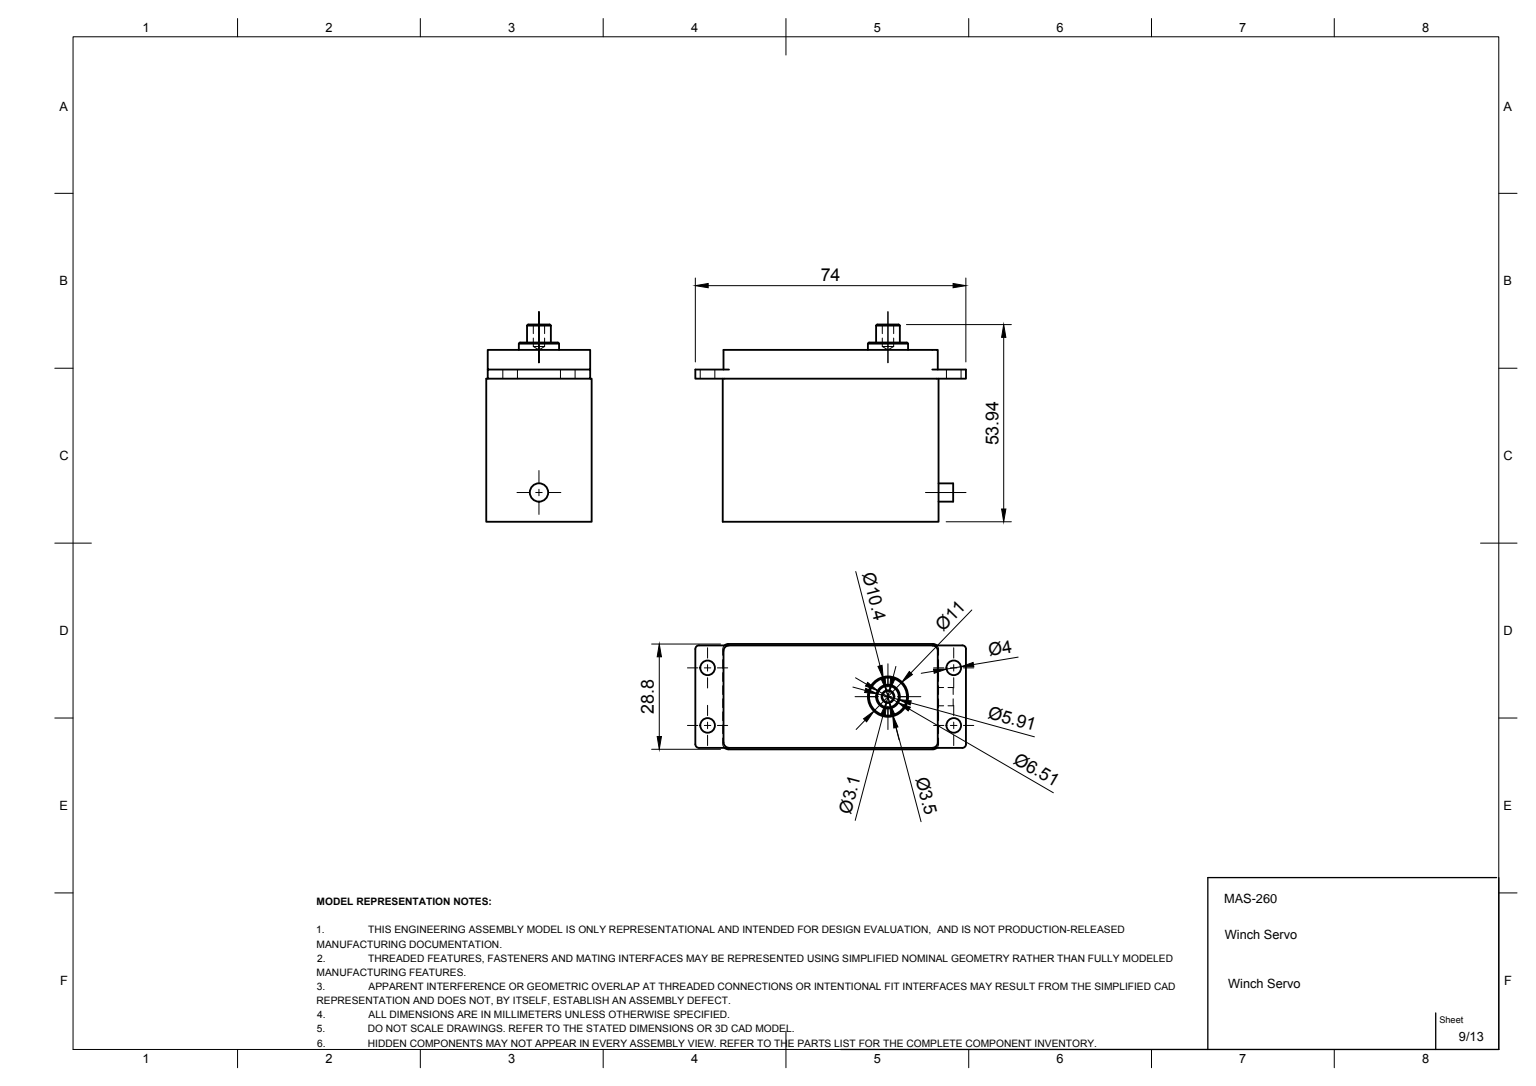
ISO-10303-21;
HEADER;
/* Generated by software containing ST-Developer
 * from STEP Tools, Inc. (www.steptools.com) 
 */

FILE_DESCRIPTION(
/* description */ (''),
/* implementation_level */ '2;1');

FILE_NAME(
/* name */ 'Winch Servo.step',
/* time_stamp */ '2026-10-15T13:29:10-07:00',
/* author */ (''),
/* organization */ (''),
/* preprocessor_version */ 'ST-DEVELOPER v20.2',
/* originating_system */ 'Autodesk Translation Framework v15.15.0.0',
/* authorisation */ '');

FILE_SCHEMA (('AUTOMOTIVE_DESIGN { 1 0 10303 214 3 1 1 }'));
ENDSEC;

DATA;
#10=MECHANICAL_DESIGN_GEOMETRIC_PRESENTATION_REPRESENTATION('',(#935),#83219);
#907=SHAPE_REPRESENTATION_RELATIONSHIP('SRR','None',#83302,#921);
#921=ADVANCED_BREP_SHAPE_REPRESENTATION('',(#949),#83207);
#935=STYLED_ITEM('',(#83381),#949);
#949=MANIFOLD_SOLID_BREP('Body1',#26931);
#1001=FACE_BOUND('',#3951,.T.);
#1002=FACE_BOUND('',#3957,.T.);
#1003=FACE_BOUND('',#3966,.T.);
#1004=FACE_BOUND('',#3968,.T.);
#1005=FACE_BOUND('',#3969,.T.);
#1006=FACE_BOUND('',#3971,.T.);
#1007=FACE_BOUND('',#3972,.T.);
#1008=FACE_BOUND('',#3974,.T.);
#1009=FACE_BOUND('',#3975,.T.);
#1010=FACE_BOUND('',#3985,.T.);
#1011=FACE_BOUND('',#3986,.T.);
#1012=FACE_BOUND('',#3993,.T.);
#1227=PLANE('',#27364);
#1228=PLANE('',#27382);
#1229=PLANE('',#27392);
#1230=PLANE('',#27395);
#1231=PLANE('',#27402);
#1232=PLANE('',#27409);
#1233=PLANE('',#27410);
#1234=PLANE('',#27413);
#1235=PLANE('',#27416);
#1236=PLANE('',#27421);
#1237=PLANE('',#27423);
#1238=PLANE('',#27426);
#1239=PLANE('',#27429);
#1240=PLANE('',#27431);
#1241=PLANE('',#27434);
#1242=PLANE('',#27437);
#1243=PLANE('',#27441);
#1244=PLANE('',#27445);
#1245=PLANE('',#27448);
#1246=PLANE('',#27451);
#1247=PLANE('',#27452);
#2173=CYLINDRICAL_SURFACE('',#27361,2.5);
#2174=CYLINDRICAL_SURFACE('',#27365,2.);
#2175=CYLINDRICAL_SURFACE('',#27368,2.);
#2176=CYLINDRICAL_SURFACE('',#27371,2.);
#2177=CYLINDRICAL_SURFACE('',#27374,2.);
#2178=CYLINDRICAL_SURFACE('',#27380,1.55);
#2179=CYLINDRICAL_SURFACE('',#27385,3.255);
#2180=CYLINDRICAL_SURFACE('',#27389,5.5);
#2181=CYLINDRICAL_SURFACE('',#27396,1.5);
#2182=CYLINDRICAL_SURFACE('',#27399,1.5);
#2183=CYLINDRICAL_SURFACE('',#27403,1.5);
#2184=CYLINDRICAL_SURFACE('',#27406,1.49999999999999);
#2185=CYLINDRICAL_SURFACE('',#27422,0.999999999999992);
#2186=CYLINDRICAL_SURFACE('',#27424,1.);
#2187=CYLINDRICAL_SURFACE('',#27427,0.999999999999999);
#2188=CYLINDRICAL_SURFACE('',#27430,0.999999999999996);
#2189=CYLINDRICAL_SURFACE('',#27438,1.5);
#2190=CYLINDRICAL_SURFACE('',#27442,1.5);
#2191=CYLINDRICAL_SURFACE('',#27446,1.5);
#2192=CYLINDRICAL_SURFACE('',#27449,1.49999999999999);
#2523=FACE_OUTER_BOUND('',#3942,.T.);
#2524=FACE_OUTER_BOUND('',#3943,.T.);
#2525=FACE_OUTER_BOUND('',#3944,.T.);
#2526=FACE_OUTER_BOUND('',#3945,.T.);
#2527=FACE_OUTER_BOUND('',#3946,.T.);
#2528=FACE_OUTER_BOUND('',#3947,.T.);
#2529=FACE_OUTER_BOUND('',#3948,.T.);
#2530=FACE_OUTER_BOUND('',#3949,.T.);
#2531=FACE_OUTER_BOUND('',#3950,.T.);
#2532=FACE_OUTER_BOUND('',#3952,.T.);
#2533=FACE_OUTER_BOUND('',#3953,.T.);
#2534=FACE_OUTER_BOUND('',#3954,.T.);
#2535=FACE_OUTER_BOUND('',#3955,.T.);
#2536=FACE_OUTER_BOUND('',#3956,.T.);
#2537=FACE_OUTER_BOUND('',#3958,.T.);
#2538=FACE_OUTER_BOUND('',#3959,.T.);
#2539=FACE_OUTER_BOUND('',#3960,.T.);
#2540=FACE_OUTER_BOUND('',#3961,.T.);
#2541=FACE_OUTER_BOUND('',#3962,.T.);
#2542=FACE_OUTER_BOUND('',#3963,.T.);
#2543=FACE_OUTER_BOUND('',#3964,.T.);
#2544=FACE_OUTER_BOUND('',#3965,.T.);
#2545=FACE_OUTER_BOUND('',#3967,.T.);
#2546=FACE_OUTER_BOUND('',#3970,.T.);
#2547=FACE_OUTER_BOUND('',#3973,.T.);
#2548=FACE_OUTER_BOUND('',#3976,.T.);
#2549=FACE_OUTER_BOUND('',#3977,.T.);
#2550=FACE_OUTER_BOUND('',#3978,.T.);
#2551=FACE_OUTER_BOUND('',#3979,.T.);
#2552=FACE_OUTER_BOUND('',#3980,.T.);
#2553=FACE_OUTER_BOUND('',#3981,.T.);
#2554=FACE_OUTER_BOUND('',#3982,.T.);
#2555=FACE_OUTER_BOUND('',#3983,.T.);
#2556=FACE_OUTER_BOUND('',#3984,.T.);
#2557=FACE_OUTER_BOUND('',#3987,.T.);
#2558=FACE_OUTER_BOUND('',#3988,.T.);
#2559=FACE_OUTER_BOUND('',#3989,.T.);
#2560=FACE_OUTER_BOUND('',#3990,.T.);
#2561=FACE_OUTER_BOUND('',#3991,.T.);
#2562=FACE_OUTER_BOUND('',#3992,.T.);
#2563=FACE_OUTER_BOUND('',#3994,.T.);
#2564=FACE_OUTER_BOUND('',#3995,.T.);
#2565=FACE_OUTER_BOUND('',#3996,.T.);
#2566=FACE_OUTER_BOUND('',#3997,.T.);
#2567=FACE_OUTER_BOUND('',#3998,.T.);
#3942=EDGE_LOOP('',(#18396,#18397,#18398,#18399));
#3943=EDGE_LOOP('',(#18400));
#3944=EDGE_LOOP('',(#18401,#18402,#18403,#18404));
#3945=EDGE_LOOP('',(#18405,#18406,#18407,#18408));
#3946=EDGE_LOOP('',(#18409,#18410,#18411,#18412));
#3947=EDGE_LOOP('',(#18413,#18414,#18415,#18416));
#3948=EDGE_LOOP('',(#18417,#18418,#18419,#18420));
#3949=EDGE_LOOP('',(#18421,#18422,#18423,#18424));
#3950=EDGE_LOOP('',(#18425));
#3951=EDGE_LOOP('',(#18426));
#3952=EDGE_LOOP('',(#18427,#18428,#18429));
#3953=EDGE_LOOP('',(#18430,#18431,#18432,#18433));
#3954=EDGE_LOOP('',(#18434,#18435,#18436,#18437));
#3955=EDGE_LOOP('',(#18438,#18439,#18440,#18441));
#3956=EDGE_LOOP('',(#18442));
#3957=EDGE_LOOP('',(#18443));
#3958=EDGE_LOOP('',(#18444,#18445,#18446,#18447));
#3959=EDGE_LOOP('',(#18448,#18449,#18450,#18451));
#3960=EDGE_LOOP('',(#18452,#18453,#18454,#18455));
#3961=EDGE_LOOP('',(#18456,#18457,#18458,#18459));
#3962=EDGE_LOOP('',(#18460,#18461,#18462,#18463));
#3963=EDGE_LOOP('',(#18464,#18465,#18466,#18467));
#3964=EDGE_LOOP('',(#18468,#18469,#18470,#18471));
#3965=EDGE_LOOP('',(#18472,#18473,#18474,#18475,#18476,#18477,#18478,#18479));
#3966=EDGE_LOOP('',(#18480));
#3967=EDGE_LOOP('',(#18481,#18482,#18483,#18484,#18485,#18486,#18487,#18488));
#3968=EDGE_LOOP('',(#18489));
#3969=EDGE_LOOP('',(#18490));
#3970=EDGE_LOOP('',(#18491,#18492,#18493,#18494,#18495,#18496,#18497,#18498));
#3971=EDGE_LOOP('',(#18499));
#3972=EDGE_LOOP('',(#18500));
#3973=EDGE_LOOP('',(#18501,#18502,#18503,#18504,#18505,#18506,#18507,#18508));
#3974=EDGE_LOOP('',(#18509));
#3975=EDGE_LOOP('',(#18510));
#3976=EDGE_LOOP('',(#18511,#18512,#18513,#18514));
#3977=EDGE_LOOP('',(#18515,#18516,#18517,#18518));
#3978=EDGE_LOOP('',(#18519,#18520,#18521,#18522,#18523,#18524,#18525,#18526,
#18527,#18528));
#3979=EDGE_LOOP('',(#18529,#18530,#18531,#18532));
#3980=EDGE_LOOP('',(#18533,#18534,#18535,#18536));
#3981=EDGE_LOOP('',(#18537,#18538,#18539,#18540));
#3982=EDGE_LOOP('',(#18541,#18542,#18543,#18544,#18545,#18546,#18547,#18548,
#18549,#18550));
#3983=EDGE_LOOP('',(#18551,#18552,#18553,#18554));
#3984=EDGE_LOOP('',(#18555,#18556,#18557,#18558,#18559,#18560,#18561,#18562));
#3985=EDGE_LOOP('',(#18563));
#3986=EDGE_LOOP('',(#18564));
#3987=EDGE_LOOP('',(#18565,#18566,#18567,#18568));
#3988=EDGE_LOOP('',(#18569,#18570,#18571,#18572));
#3989=EDGE_LOOP('',(#18573,#18574,#18575,#18576,#18577));
#3990=EDGE_LOOP('',(#18578,#18579,#18580,#18581));
#3991=EDGE_LOOP('',(#18582,#18583,#18584,#18585,#18586));
#3992=EDGE_LOOP('',(#18587,#18588,#18589,#18590));
#3993=EDGE_LOOP('',(#18591));
#3994=EDGE_LOOP('',(#18592,#18593,#18594,#18595,#18596));
#3995=EDGE_LOOP('',(#18597,#18598,#18599,#18600));
#3996=EDGE_LOOP('',(#18601,#18602,#18603,#18604,#18605));
#3997=EDGE_LOOP('',(#18606,#18607,#18608,#18609));
#3998=EDGE_LOOP('',(#18610,#18611,#18612,#18613,#18614,#18615,#18616,#18617));
#5589=LINE('',#36906,#8100);
#5590=LINE('',#36913,#8101);
#5591=LINE('',#36919,#8102);
#5592=LINE('',#36925,#8103);
#5593=LINE('',#36931,#8104);
#5594=LINE('',#36937,#8105);
#5595=LINE('',#36941,#8106);
#5596=LINE('',#36948,#8107);
#5597=LINE('',#36953,#8108);
#5598=LINE('',#36956,#8109);
#5599=LINE('',#36961,#8110);
#5600=LINE('',#36967,#8111);
#5601=LINE('',#36971,#8112);
#5602=LINE('',#36973,#8113);
#5603=LINE('',#36975,#8114);
#5604=LINE('',#36976,#8115);
#5605=LINE('',#36982,#8116);
#5606=LINE('',#36988,#8117);
#5607=LINE('',#36991,#8118);
#5608=LINE('',#36994,#8119);
#5609=LINE('',#36996,#8120);
#5610=LINE('',#36997,#8121);
#5611=LINE('',#37003,#8122);
#5612=LINE('',#37008,#8123);
#5613=LINE('',#37011,#8124);
#5614=LINE('',#37012,#8125);
#5615=LINE('',#37015,#8126);
#5616=LINE('',#37019,#8127);
#5617=LINE('',#37022,#8128);
#5618=LINE('',#37025,#8129);
#5619=LINE('',#37029,#8130);
#5620=LINE('',#37032,#8131);
#5621=LINE('',#37038,#8132);
#5622=LINE('',#37042,#8133);
#5623=LINE('',#37046,#8134);
#5624=LINE('',#37049,#8135);
#5625=LINE('',#37051,#8136);
#5626=LINE('',#37052,#8137);
#5627=LINE('',#37054,#8138);
#5628=LINE('',#37057,#8139);
#5629=LINE('',#37059,#8140);
#5630=LINE('',#37060,#8141);
#5631=LINE('',#37064,#8142);
#5632=LINE('',#37067,#8143);
#5633=LINE('',#37068,#8144);
#5634=LINE('',#37072,#8145);
#5635=LINE('',#37075,#8146);
#5636=LINE('',#37076,#8147);
#5637=LINE('',#37077,#8148);
#5638=LINE('',#37084,#8149);
#5639=LINE('',#37089,#8150);
#5640=LINE('',#37094,#8151);
#5641=LINE('',#37095,#8152);
#5642=LINE('',#37096,#8153);
#5643=LINE('',#37102,#8154);
#5644=LINE('',#37105,#8155);
#5645=LINE('',#37107,#8156);
#5646=LINE('',#37108,#8157);
#5647=LINE('',#37113,#8158);
#5648=LINE('',#37116,#8159);
#5649=LINE('',#37117,#8160);
#5650=LINE('',#37121,#8161);
#5651=LINE('',#37124,#8162);
#5652=LINE('',#37125,#8163);
#8100=VECTOR('',#30097,2.5);
#8101=VECTOR('',#30106,2.);
#8102=VECTOR('',#30113,2.);
#8103=VECTOR('',#30120,2.);
#8104=VECTOR('',#30127,2.);
#8105=VECTOR('',#30134,1.65);
#8106=VECTOR('',#30139,1.55);
#8107=VECTOR('',#30148,1.55);
#8108=VECTOR('',#30153,3.255);
#8109=VECTOR('',#30158,3.105);
#8110=VECTOR('',#30163,5.5);
#8111=VECTOR('',#30172,5.35);
#8112=VECTOR('',#30175,10.);
#8113=VECTOR('',#30176,10.);
#8114=VECTOR('',#30177,10.);
#8115=VECTOR('',#30178,10.);
#8116=VECTOR('',#30185,10.);
#8117=VECTOR('',#30190,10.);
#8118=VECTOR('',#30193,10.);
#8119=VECTOR('',#30196,10.);
#8120=VECTOR('',#30197,10.);
#8121=VECTOR('',#30198,10.);
#8122=VECTOR('',#30205,10.);
#8123=VECTOR('',#30210,10.);
#8124=VECTOR('',#30215,10.);
#8125=VECTOR('',#30216,10.);
#8126=VECTOR('',#30219,10.);
#8127=VECTOR('',#30222,10.);
#8128=VECTOR('',#30225,10.);
#8129=VECTOR('',#30228,10.);
#8130=VECTOR('',#30231,10.);
#8131=VECTOR('',#30234,10.);
#8132=VECTOR('',#30239,10.);
#8133=VECTOR('',#30242,10.);
#8134=VECTOR('',#30245,10.);
#8135=VECTOR('',#30248,10.);
#8136=VECTOR('',#30251,10.);
#8137=VECTOR('',#30252,10.);
#8138=VECTOR('',#30255,10.);
#8139=VECTOR('',#30258,10.);
#8140=VECTOR('',#30259,10.);
#8141=VECTOR('',#30260,10.);
#8142=VECTOR('',#30265,10.);
#8143=VECTOR('',#30268,10.);
#8144=VECTOR('',#30269,10.);
#8145=VECTOR('',#30274,10.);
#8146=VECTOR('',#30277,10.);
#8147=VECTOR('',#30278,10.);
#8148=VECTOR('',#30279,10.);
#8149=VECTOR('',#30288,10.);
#8150=VECTOR('',#30293,10.);
#8151=VECTOR('',#30298,10.);
#8152=VECTOR('',#30299,10.);
#8153=VECTOR('',#30300,10.);
#8154=VECTOR('',#30307,10.);
#8155=VECTOR('',#30310,10.);
#8156=VECTOR('',#30311,10.);
#8157=VECTOR('',#30312,10.);
#8158=VECTOR('',#30319,10.);
#8159=VECTOR('',#30322,10.);
#8160=VECTOR('',#30323,10.);
#8161=VECTOR('',#30328,10.);
#8162=VECTOR('',#30331,10.);
#8163=VECTOR('',#30332,10.);
#10392=CIRCLE('',#27362,2.5);
#10393=CIRCLE('',#27363,2.5);
#10394=CIRCLE('',#27366,2.);
#10395=CIRCLE('',#27367,2.);
#10396=CIRCLE('',#27369,2.);
#10397=CIRCLE('',#27370,2.);
#10398=CIRCLE('',#27372,2.);
#10399=CIRCLE('',#27373,2.);
#10400=CIRCLE('',#27375,2.);
#10401=CIRCLE('',#27376,2.);
#10402=CIRCLE('',#27378,1.55);
#10403=CIRCLE('',#27379,1.75);
#10404=CIRCLE('',#27381,1.55);
#10405=CIRCLE('',#27383,2.955);
#10406=CIRCLE('',#27386,3.255);
#10407=CIRCLE('',#27387,3.255);
#10408=CIRCLE('',#27390,5.5);
#10409=CIRCLE('',#27391,5.5);
#10410=CIRCLE('',#27393,5.2);
#10411=CIRCLE('',#27397,1.5);
#10412=CIRCLE('',#27398,1.5);
#10413=CIRCLE('',#27400,1.5);
#10414=CIRCLE('',#27401,1.5);
#10415=CIRCLE('',#27404,1.5);
#10416=CIRCLE('',#27405,1.5);
#10417=CIRCLE('',#27407,1.49999999999999);
#10418=CIRCLE('',#27408,1.49999999999999);
#10419=CIRCLE('',#27411,0.999999999999992);
#10420=CIRCLE('',#27412,0.999999999999996);
#10421=CIRCLE('',#27414,0.999999999999999);
#10422=CIRCLE('',#27415,1.);
#10423=CIRCLE('',#27417,1.5);
#10424=CIRCLE('',#27418,1.49999999999999);
#10425=CIRCLE('',#27419,0.999999999999996);
#10426=CIRCLE('',#27420,0.999999999999992);
#10427=CIRCLE('',#27425,1.);
#10428=CIRCLE('',#27428,0.999999999999999);
#10429=CIRCLE('',#27432,1.5);
#10430=CIRCLE('',#27433,1.5);
#10431=CIRCLE('',#27435,1.49999999999999);
#10432=CIRCLE('',#27436,1.5);
#10433=CIRCLE('',#27439,1.5);
#10434=CIRCLE('',#27440,1.5);
#10435=CIRCLE('',#27443,1.5);
#10436=CIRCLE('',#27444,1.5);
#10437=CIRCLE('',#27447,1.5);
#10438=CIRCLE('',#27450,1.49999999999999);
#11298=VERTEX_POINT('',#36903);
#11299=VERTEX_POINT('',#36905);
#11300=VERTEX_POINT('',#36910);
#11301=VERTEX_POINT('',#36912);
#11302=VERTEX_POINT('',#36916);
#11303=VERTEX_POINT('',#36918);
#11304=VERTEX_POINT('',#36922);
#11305=VERTEX_POINT('',#36924);
#11306=VERTEX_POINT('',#36928);
#11307=VERTEX_POINT('',#36930);
#11308=VERTEX_POINT('',#36934);
#11309=VERTEX_POINT('',#36936);
#11310=VERTEX_POINT('',#36940);
#11311=VERTEX_POINT('',#36944);
#11312=VERTEX_POINT('',#36947);
#11313=VERTEX_POINT('',#36950);
#11314=VERTEX_POINT('',#36952);
#11315=VERTEX_POINT('',#36958);
#11316=VERTEX_POINT('',#36960);
#11317=VERTEX_POINT('',#36964);
#11318=VERTEX_POINT('',#36969);
#11319=VERTEX_POINT('',#36970);
#11320=VERTEX_POINT('',#36972);
#11321=VERTEX_POINT('',#36974);
#11322=VERTEX_POINT('',#36978);
#11323=VERTEX_POINT('',#36980);
#11324=VERTEX_POINT('',#36984);
#11325=VERTEX_POINT('',#36985);
#11326=VERTEX_POINT('',#36987);
#11327=VERTEX_POINT('',#36989);
#11328=VERTEX_POINT('',#36993);
#11329=VERTEX_POINT('',#36995);
#11330=VERTEX_POINT('',#36999);
#11331=VERTEX_POINT('',#37001);
#11332=VERTEX_POINT('',#37005);
#11333=VERTEX_POINT('',#37007);
#11334=VERTEX_POINT('',#37014);
#11335=VERTEX_POINT('',#37016);
#11336=VERTEX_POINT('',#37018);
#11337=VERTEX_POINT('',#37020);
#11338=VERTEX_POINT('',#37024);
#11339=VERTEX_POINT('',#37026);
#11340=VERTEX_POINT('',#37028);
#11341=VERTEX_POINT('',#37030);
#11342=VERTEX_POINT('',#37034);
#11343=VERTEX_POINT('',#37035);
#11344=VERTEX_POINT('',#37037);
#11345=VERTEX_POINT('',#37039);
#11346=VERTEX_POINT('',#37041);
#11347=VERTEX_POINT('',#37043);
#11348=VERTEX_POINT('',#37045);
#11349=VERTEX_POINT('',#37047);
#11350=VERTEX_POINT('',#37056);
#11351=VERTEX_POINT('',#37058);
#11352=VERTEX_POINT('',#37062);
#11353=VERTEX_POINT('',#37066);
#11354=VERTEX_POINT('',#37070);
#11355=VERTEX_POINT('',#37074);
#11356=VERTEX_POINT('',#37080);
#11357=VERTEX_POINT('',#37082);
#11358=VERTEX_POINT('',#37086);
#11359=VERTEX_POINT('',#37088);
#11360=VERTEX_POINT('',#37092);
#11361=VERTEX_POINT('',#37093);
#11362=VERTEX_POINT('',#37098);
#11363=VERTEX_POINT('',#37100);
#11364=VERTEX_POINT('',#37104);
#11365=VERTEX_POINT('',#37106);
#11366=VERTEX_POINT('',#37110);
#11367=VERTEX_POINT('',#37115);
#11368=VERTEX_POINT('',#37119);
#11369=VERTEX_POINT('',#37123);
#14059=EDGE_CURVE('',#11298,#11298,#10392,.T.);
#14060=EDGE_CURVE('',#11298,#11299,#5589,.T.);
#14061=EDGE_CURVE('',#11299,#11299,#10393,.T.);
#14062=EDGE_CURVE('',#11300,#11300,#10394,.T.);
#14063=EDGE_CURVE('',#11300,#11301,#5590,.T.);
#14064=EDGE_CURVE('',#11301,#11301,#10395,.T.);
#14065=EDGE_CURVE('',#11302,#11302,#10396,.T.);
#14066=EDGE_CURVE('',#11302,#11303,#5591,.T.);
#14067=EDGE_CURVE('',#11303,#11303,#10397,.T.);
#14068=EDGE_CURVE('',#11304,#11304,#10398,.T.);
#14069=EDGE_CURVE('',#11304,#11305,#5592,.T.);
#14070=EDGE_CURVE('',#11305,#11305,#10399,.T.);
#14071=EDGE_CURVE('',#11306,#11306,#10400,.T.);
#14072=EDGE_CURVE('',#11306,#11307,#5593,.T.);
#14073=EDGE_CURVE('',#11307,#11307,#10401,.T.);
#14074=EDGE_CURVE('',#11308,#11308,#10402,.T.);
#14075=EDGE_CURVE('',#11308,#11309,#5594,.T.);
#14076=EDGE_CURVE('',#11309,#11309,#10403,.T.);
#14077=EDGE_CURVE('',#11308,#11310,#5595,.T.);
#14078=EDGE_CURVE('',#11310,#11310,#10404,.T.);
#14079=EDGE_CURVE('',#11311,#11311,#10405,.T.);
#14080=EDGE_CURVE('',#11312,#11310,#5596,.T.);
#14081=EDGE_CURVE('',#11313,#11313,#10406,.T.);
#14082=EDGE_CURVE('',#11313,#11314,#5597,.T.);
#14083=EDGE_CURVE('',#11314,#11314,#10407,.T.);
#14084=EDGE_CURVE('',#11314,#11311,#5598,.T.);
#14085=EDGE_CURVE('',#11315,#11315,#10408,.T.);
#14086=EDGE_CURVE('',#11315,#11316,#5599,.T.);
#14087=EDGE_CURVE('',#11316,#11316,#10409,.T.);
#14088=EDGE_CURVE('',#11317,#11317,#10410,.T.);
#14089=EDGE_CURVE('',#11316,#11317,#5600,.T.);
#14090=EDGE_CURVE('',#11318,#11319,#5601,.T.);
#14091=EDGE_CURVE('',#11318,#11320,#5602,.T.);
#14092=EDGE_CURVE('',#11321,#11320,#5603,.T.);
#14093=EDGE_CURVE('',#11319,#11321,#5604,.T.);
#14094=EDGE_CURVE('',#11319,#11322,#10411,.T.);
#14095=EDGE_CURVE('',#11323,#11321,#10412,.T.);
#14096=EDGE_CURVE('',#11322,#11323,#5605,.T.);
#14097=EDGE_CURVE('',#11324,#11325,#10413,.T.);
#14098=EDGE_CURVE('',#11324,#11326,#5606,.T.);
#14099=EDGE_CURVE('',#11327,#11326,#10414,.T.);
#14100=EDGE_CURVE('',#11325,#11327,#5607,.T.);
#14101=EDGE_CURVE('',#11325,#11328,#5608,.T.);
#14102=EDGE_CURVE('',#11329,#11327,#5609,.T.);
#14103=EDGE_CURVE('',#11328,#11329,#5610,.T.);
#14104=EDGE_CURVE('',#11328,#11330,#10415,.T.);
#14105=EDGE_CURVE('',#11331,#11329,#10416,.T.);
#14106=EDGE_CURVE('',#11330,#11331,#5611,.T.);
#14107=EDGE_CURVE('',#11332,#11318,#10417,.T.);
#14108=EDGE_CURVE('',#11332,#11333,#5612,.T.);
#14109=EDGE_CURVE('',#11320,#11333,#10418,.T.);
#14110=EDGE_CURVE('',#11333,#11331,#5613,.T.);
#14111=EDGE_CURVE('',#11326,#11323,#5614,.T.);
#14112=EDGE_CURVE('',#11322,#11334,#5615,.T.);
#14113=EDGE_CURVE('',#11334,#11335,#10419,.T.);
#14114=EDGE_CURVE('',#11335,#11336,#5616,.T.);
#14115=EDGE_CURVE('',#11336,#11337,#10420,.T.);
#14116=EDGE_CURVE('',#11337,#11332,#5617,.T.);
#14117=EDGE_CURVE('',#11330,#11338,#5618,.T.);
#14118=EDGE_CURVE('',#11338,#11339,#10421,.T.);
#14119=EDGE_CURVE('',#11339,#11340,#5619,.T.);
#14120=EDGE_CURVE('',#11340,#11341,#10422,.T.);
#14121=EDGE_CURVE('',#11341,#11324,#5620,.T.);
#14122=EDGE_CURVE('',#11342,#11343,#10423,.T.);
#14123=EDGE_CURVE('',#11343,#11344,#5621,.T.);
#14124=EDGE_CURVE('',#11344,#11345,#10424,.T.);
#14125=EDGE_CURVE('',#11345,#11346,#5622,.T.);
#14126=EDGE_CURVE('',#11347,#11346,#10425,.T.);
#14127=EDGE_CURVE('',#11347,#11348,#5623,.T.);
#14128=EDGE_CURVE('',#11349,#11348,#10426,.T.);
#14129=EDGE_CURVE('',#11349,#11342,#5624,.T.);
#14130=EDGE_CURVE('',#11347,#11336,#5625,.T.);
#14131=EDGE_CURVE('',#11348,#11335,#5626,.T.);
#14132=EDGE_CURVE('',#11349,#11334,#5627,.T.);
#14133=EDGE_CURVE('',#11350,#11341,#5628,.T.);
#14134=EDGE_CURVE('',#11351,#11350,#5629,.T.);
#14135=EDGE_CURVE('',#11342,#11351,#5630,.T.);
#14136=EDGE_CURVE('',#11352,#11350,#10427,.T.);
#14137=EDGE_CURVE('',#11352,#11340,#5631,.T.);
#14138=EDGE_CURVE('',#11352,#11353,#5632,.T.);
#14139=EDGE_CURVE('',#11353,#11339,#5633,.T.);
#14140=EDGE_CURVE('',#11354,#11353,#10428,.T.);
#14141=EDGE_CURVE('',#11354,#11338,#5634,.T.);
#14142=EDGE_CURVE('',#11354,#11355,#5635,.T.);
#14143=EDGE_CURVE('',#11346,#11337,#5636,.T.);
#14144=EDGE_CURVE('',#11355,#11345,#5637,.T.);
#14145=EDGE_CURVE('',#11356,#11351,#10429,.T.);
#14146=EDGE_CURVE('',#11355,#11357,#10430,.T.);
#14147=EDGE_CURVE('',#11357,#11356,#5638,.T.);
#14148=EDGE_CURVE('',#11345,#11358,#10431,.T.);
#14149=EDGE_CURVE('',#11358,#11359,#5639,.T.);
#14150=EDGE_CURVE('',#11359,#11355,#10432,.T.);
#14151=EDGE_CURVE('',#11360,#11361,#5640,.T.);
#14152=EDGE_CURVE('',#11360,#11344,#5641,.T.);
#14153=EDGE_CURVE('',#11361,#11343,#5642,.T.);
#14154=EDGE_CURVE('',#11362,#11361,#10433,.T.);
#14155=EDGE_CURVE('',#11363,#11342,#10434,.T.);
#14156=EDGE_CURVE('',#11362,#11363,#5643,.T.);
#14157=EDGE_CURVE('',#11362,#11364,#5644,.T.);
#14158=EDGE_CURVE('',#11365,#11363,#5645,.T.);
#14159=EDGE_CURVE('',#11364,#11365,#5646,.T.);
#14160=EDGE_CURVE('',#11366,#11364,#10435,.T.);
#14161=EDGE_CURVE('',#11351,#11365,#10436,.T.);
#14162=EDGE_CURVE('',#11366,#11356,#5647,.T.);
#14163=EDGE_CURVE('',#11366,#11367,#5648,.T.);
#14164=EDGE_CURVE('',#11367,#11357,#5649,.T.);
#14165=EDGE_CURVE('',#11368,#11367,#10437,.T.);
#14166=EDGE_CURVE('',#11368,#11359,#5650,.T.);
#14167=EDGE_CURVE('',#11368,#11369,#5651,.T.);
#14168=EDGE_CURVE('',#11369,#11358,#5652,.T.);
#14169=EDGE_CURVE('',#11360,#11369,#10438,.T.);
#18396=ORIENTED_EDGE('',*,*,#14059,.F.);
#18397=ORIENTED_EDGE('',*,*,#14060,.T.);
#18398=ORIENTED_EDGE('',*,*,#14061,.F.);
#18399=ORIENTED_EDGE('',*,*,#14060,.F.);
#18400=ORIENTED_EDGE('',*,*,#14059,.T.);
#18401=ORIENTED_EDGE('',*,*,#14062,.F.);
#18402=ORIENTED_EDGE('',*,*,#14063,.T.);
#18403=ORIENTED_EDGE('',*,*,#14064,.F.);
#18404=ORIENTED_EDGE('',*,*,#14063,.F.);
#18405=ORIENTED_EDGE('',*,*,#14065,.F.);
#18406=ORIENTED_EDGE('',*,*,#14066,.T.);
#18407=ORIENTED_EDGE('',*,*,#14067,.F.);
#18408=ORIENTED_EDGE('',*,*,#14066,.F.);
#18409=ORIENTED_EDGE('',*,*,#14068,.F.);
#18410=ORIENTED_EDGE('',*,*,#14069,.T.);
#18411=ORIENTED_EDGE('',*,*,#14070,.F.);
#18412=ORIENTED_EDGE('',*,*,#14069,.F.);
#18413=ORIENTED_EDGE('',*,*,#14071,.F.);
#18414=ORIENTED_EDGE('',*,*,#14072,.T.);
#18415=ORIENTED_EDGE('',*,*,#14073,.F.);
#18416=ORIENTED_EDGE('',*,*,#14072,.F.);
#18417=ORIENTED_EDGE('',*,*,#14074,.T.);
#18418=ORIENTED_EDGE('',*,*,#14075,.T.);
#18419=ORIENTED_EDGE('',*,*,#14076,.T.);
#18420=ORIENTED_EDGE('',*,*,#14075,.F.);
#18421=ORIENTED_EDGE('',*,*,#14074,.F.);
#18422=ORIENTED_EDGE('',*,*,#14077,.T.);
#18423=ORIENTED_EDGE('',*,*,#14078,.T.);
#18424=ORIENTED_EDGE('',*,*,#14077,.F.);
#18425=ORIENTED_EDGE('',*,*,#14079,.F.);
#18426=ORIENTED_EDGE('',*,*,#14076,.F.);
#18427=ORIENTED_EDGE('',*,*,#14080,.T.);
#18428=ORIENTED_EDGE('',*,*,#14078,.F.);
#18429=ORIENTED_EDGE('',*,*,#14080,.F.);
#18430=ORIENTED_EDGE('',*,*,#14081,.F.);
#18431=ORIENTED_EDGE('',*,*,#14082,.T.);
#18432=ORIENTED_EDGE('',*,*,#14083,.T.);
#18433=ORIENTED_EDGE('',*,*,#14082,.F.);
#18434=ORIENTED_EDGE('',*,*,#14083,.F.);
#18435=ORIENTED_EDGE('',*,*,#14084,.T.);
#18436=ORIENTED_EDGE('',*,*,#14079,.T.);
#18437=ORIENTED_EDGE('',*,*,#14084,.F.);
#18438=ORIENTED_EDGE('',*,*,#14085,.F.);
#18439=ORIENTED_EDGE('',*,*,#14086,.T.);
#18440=ORIENTED_EDGE('',*,*,#14087,.T.);
#18441=ORIENTED_EDGE('',*,*,#14086,.F.);
#18442=ORIENTED_EDGE('',*,*,#14088,.F.);
#18443=ORIENTED_EDGE('',*,*,#14081,.T.);
#18444=ORIENTED_EDGE('',*,*,#14087,.F.);
#18445=ORIENTED_EDGE('',*,*,#14089,.T.);
#18446=ORIENTED_EDGE('',*,*,#14088,.T.);
#18447=ORIENTED_EDGE('',*,*,#14089,.F.);
#18448=ORIENTED_EDGE('',*,*,#14090,.F.);
#18449=ORIENTED_EDGE('',*,*,#14091,.T.);
#18450=ORIENTED_EDGE('',*,*,#14092,.F.);
#18451=ORIENTED_EDGE('',*,*,#14093,.F.);
#18452=ORIENTED_EDGE('',*,*,#14094,.F.);
#18453=ORIENTED_EDGE('',*,*,#14093,.T.);
#18454=ORIENTED_EDGE('',*,*,#14095,.F.);
#18455=ORIENTED_EDGE('',*,*,#14096,.F.);
#18456=ORIENTED_EDGE('',*,*,#14097,.F.);
#18457=ORIENTED_EDGE('',*,*,#14098,.T.);
#18458=ORIENTED_EDGE('',*,*,#14099,.F.);
#18459=ORIENTED_EDGE('',*,*,#14100,.F.);
#18460=ORIENTED_EDGE('',*,*,#14101,.F.);
#18461=ORIENTED_EDGE('',*,*,#14100,.T.);
#18462=ORIENTED_EDGE('',*,*,#14102,.F.);
#18463=ORIENTED_EDGE('',*,*,#14103,.F.);
#18464=ORIENTED_EDGE('',*,*,#14104,.F.);
#18465=ORIENTED_EDGE('',*,*,#14103,.T.);
#18466=ORIENTED_EDGE('',*,*,#14105,.F.);
#18467=ORIENTED_EDGE('',*,*,#14106,.F.);
#18468=ORIENTED_EDGE('',*,*,#14107,.F.);
#18469=ORIENTED_EDGE('',*,*,#14108,.T.);
#18470=ORIENTED_EDGE('',*,*,#14109,.F.);
#18471=ORIENTED_EDGE('',*,*,#14091,.F.);
#18472=ORIENTED_EDGE('',*,*,#14109,.T.);
#18473=ORIENTED_EDGE('',*,*,#14110,.T.);
#18474=ORIENTED_EDGE('',*,*,#14105,.T.);
#18475=ORIENTED_EDGE('',*,*,#14102,.T.);
#18476=ORIENTED_EDGE('',*,*,#14099,.T.);
#18477=ORIENTED_EDGE('',*,*,#14111,.T.);
#18478=ORIENTED_EDGE('',*,*,#14095,.T.);
#18479=ORIENTED_EDGE('',*,*,#14092,.T.);
#18480=ORIENTED_EDGE('',*,*,#14085,.T.);
#18481=ORIENTED_EDGE('',*,*,#14094,.T.);
#18482=ORIENTED_EDGE('',*,*,#14112,.T.);
#18483=ORIENTED_EDGE('',*,*,#14113,.T.);
#18484=ORIENTED_EDGE('',*,*,#14114,.T.);
#18485=ORIENTED_EDGE('',*,*,#14115,.T.);
#18486=ORIENTED_EDGE('',*,*,#14116,.T.);
#18487=ORIENTED_EDGE('',*,*,#14107,.T.);
#18488=ORIENTED_EDGE('',*,*,#14090,.T.);
#18489=ORIENTED_EDGE('',*,*,#14062,.T.);
#18490=ORIENTED_EDGE('',*,*,#14071,.T.);
#18491=ORIENTED_EDGE('',*,*,#14097,.T.);
#18492=ORIENTED_EDGE('',*,*,#14101,.T.);
#18493=ORIENTED_EDGE('',*,*,#14104,.T.);
#18494=ORIENTED_EDGE('',*,*,#14117,.T.);
#18495=ORIENTED_EDGE('',*,*,#14118,.T.);
#18496=ORIENTED_EDGE('',*,*,#14119,.T.);
#18497=ORIENTED_EDGE('',*,*,#14120,.T.);
#18498=ORIENTED_EDGE('',*,*,#14121,.T.);
#18499=ORIENTED_EDGE('',*,*,#14065,.T.);
#18500=ORIENTED_EDGE('',*,*,#14068,.T.);
#18501=ORIENTED_EDGE('',*,*,#14122,.T.);
#18502=ORIENTED_EDGE('',*,*,#14123,.T.);
#18503=ORIENTED_EDGE('',*,*,#14124,.T.);
#18504=ORIENTED_EDGE('',*,*,#14125,.T.);
#18505=ORIENTED_EDGE('',*,*,#14126,.F.);
#18506=ORIENTED_EDGE('',*,*,#14127,.T.);
#18507=ORIENTED_EDGE('',*,*,#14128,.F.);
#18508=ORIENTED_EDGE('',*,*,#14129,.T.);
#18509=ORIENTED_EDGE('',*,*,#14064,.T.);
#18510=ORIENTED_EDGE('',*,*,#14073,.T.);
#18511=ORIENTED_EDGE('',*,*,#14127,.F.);
#18512=ORIENTED_EDGE('',*,*,#14130,.T.);
#18513=ORIENTED_EDGE('',*,*,#14114,.F.);
#18514=ORIENTED_EDGE('',*,*,#14131,.F.);
#18515=ORIENTED_EDGE('',*,*,#14128,.T.);
#18516=ORIENTED_EDGE('',*,*,#14131,.T.);
#18517=ORIENTED_EDGE('',*,*,#14113,.F.);
#18518=ORIENTED_EDGE('',*,*,#14132,.F.);
#18519=ORIENTED_EDGE('',*,*,#14129,.F.);
#18520=ORIENTED_EDGE('',*,*,#14132,.T.);
#18521=ORIENTED_EDGE('',*,*,#14112,.F.);
#18522=ORIENTED_EDGE('',*,*,#14096,.T.);
#18523=ORIENTED_EDGE('',*,*,#14111,.F.);
#18524=ORIENTED_EDGE('',*,*,#14098,.F.);
#18525=ORIENTED_EDGE('',*,*,#14121,.F.);
#18526=ORIENTED_EDGE('',*,*,#14133,.F.);
#18527=ORIENTED_EDGE('',*,*,#14134,.F.);
#18528=ORIENTED_EDGE('',*,*,#14135,.F.);
#18529=ORIENTED_EDGE('',*,*,#14136,.T.);
#18530=ORIENTED_EDGE('',*,*,#14133,.T.);
#18531=ORIENTED_EDGE('',*,*,#14120,.F.);
#18532=ORIENTED_EDGE('',*,*,#14137,.F.);
#18533=ORIENTED_EDGE('',*,*,#14138,.F.);
#18534=ORIENTED_EDGE('',*,*,#14137,.T.);
#18535=ORIENTED_EDGE('',*,*,#14119,.F.);
#18536=ORIENTED_EDGE('',*,*,#14139,.F.);
#18537=ORIENTED_EDGE('',*,*,#14140,.T.);
#18538=ORIENTED_EDGE('',*,*,#14139,.T.);
#18539=ORIENTED_EDGE('',*,*,#14118,.F.);
#18540=ORIENTED_EDGE('',*,*,#14141,.F.);
#18541=ORIENTED_EDGE('',*,*,#14142,.F.);
#18542=ORIENTED_EDGE('',*,*,#14141,.T.);
#18543=ORIENTED_EDGE('',*,*,#14117,.F.);
#18544=ORIENTED_EDGE('',*,*,#14106,.T.);
#18545=ORIENTED_EDGE('',*,*,#14110,.F.);
#18546=ORIENTED_EDGE('',*,*,#14108,.F.);
#18547=ORIENTED_EDGE('',*,*,#14116,.F.);
#18548=ORIENTED_EDGE('',*,*,#14143,.F.);
#18549=ORIENTED_EDGE('',*,*,#14125,.F.);
#18550=ORIENTED_EDGE('',*,*,#14144,.F.);
#18551=ORIENTED_EDGE('',*,*,#14126,.T.);
#18552=ORIENTED_EDGE('',*,*,#14143,.T.);
#18553=ORIENTED_EDGE('',*,*,#14115,.F.);
#18554=ORIENTED_EDGE('',*,*,#14130,.F.);
#18555=ORIENTED_EDGE('',*,*,#14145,.T.);
#18556=ORIENTED_EDGE('',*,*,#14134,.T.);
#18557=ORIENTED_EDGE('',*,*,#14136,.F.);
#18558=ORIENTED_EDGE('',*,*,#14138,.T.);
#18559=ORIENTED_EDGE('',*,*,#14140,.F.);
#18560=ORIENTED_EDGE('',*,*,#14142,.T.);
#18561=ORIENTED_EDGE('',*,*,#14146,.T.);
#18562=ORIENTED_EDGE('',*,*,#14147,.T.);
#18563=ORIENTED_EDGE('',*,*,#14067,.T.);
#18564=ORIENTED_EDGE('',*,*,#14070,.T.);
#18565=ORIENTED_EDGE('',*,*,#14144,.T.);
#18566=ORIENTED_EDGE('',*,*,#14148,.T.);
#18567=ORIENTED_EDGE('',*,*,#14149,.T.);
#18568=ORIENTED_EDGE('',*,*,#14150,.T.);
#18569=ORIENTED_EDGE('',*,*,#14151,.F.);
#18570=ORIENTED_EDGE('',*,*,#14152,.T.);
#18571=ORIENTED_EDGE('',*,*,#14123,.F.);
#18572=ORIENTED_EDGE('',*,*,#14153,.F.);
#18573=ORIENTED_EDGE('',*,*,#14154,.T.);
#18574=ORIENTED_EDGE('',*,*,#14153,.T.);
#18575=ORIENTED_EDGE('',*,*,#14122,.F.);
#18576=ORIENTED_EDGE('',*,*,#14155,.F.);
#18577=ORIENTED_EDGE('',*,*,#14156,.F.);
#18578=ORIENTED_EDGE('',*,*,#14157,.F.);
#18579=ORIENTED_EDGE('',*,*,#14156,.T.);
#18580=ORIENTED_EDGE('',*,*,#14158,.F.);
#18581=ORIENTED_EDGE('',*,*,#14159,.F.);
#18582=ORIENTED_EDGE('',*,*,#14160,.T.);
#18583=ORIENTED_EDGE('',*,*,#14159,.T.);
#18584=ORIENTED_EDGE('',*,*,#14161,.F.);
#18585=ORIENTED_EDGE('',*,*,#14145,.F.);
#18586=ORIENTED_EDGE('',*,*,#14162,.F.);
#18587=ORIENTED_EDGE('',*,*,#14163,.F.);
#18588=ORIENTED_EDGE('',*,*,#14162,.T.);
#18589=ORIENTED_EDGE('',*,*,#14147,.F.);
#18590=ORIENTED_EDGE('',*,*,#14164,.F.);
#18591=ORIENTED_EDGE('',*,*,#14061,.T.);
#18592=ORIENTED_EDGE('',*,*,#14165,.T.);
#18593=ORIENTED_EDGE('',*,*,#14164,.T.);
#18594=ORIENTED_EDGE('',*,*,#14146,.F.);
#18595=ORIENTED_EDGE('',*,*,#14150,.F.);
#18596=ORIENTED_EDGE('',*,*,#14166,.F.);
#18597=ORIENTED_EDGE('',*,*,#14167,.F.);
#18598=ORIENTED_EDGE('',*,*,#14166,.T.);
#18599=ORIENTED_EDGE('',*,*,#14149,.F.);
#18600=ORIENTED_EDGE('',*,*,#14168,.F.);
#18601=ORIENTED_EDGE('',*,*,#14169,.T.);
#18602=ORIENTED_EDGE('',*,*,#14168,.T.);
#18603=ORIENTED_EDGE('',*,*,#14148,.F.);
#18604=ORIENTED_EDGE('',*,*,#14124,.F.);
#18605=ORIENTED_EDGE('',*,*,#14152,.F.);
#18606=ORIENTED_EDGE('',*,*,#14135,.T.);
#18607=ORIENTED_EDGE('',*,*,#14161,.T.);
#18608=ORIENTED_EDGE('',*,*,#14158,.T.);
#18609=ORIENTED_EDGE('',*,*,#14155,.T.);
#18610=ORIENTED_EDGE('',*,*,#14169,.F.);
#18611=ORIENTED_EDGE('',*,*,#14151,.T.);
#18612=ORIENTED_EDGE('',*,*,#14154,.F.);
#18613=ORIENTED_EDGE('',*,*,#14157,.T.);
#18614=ORIENTED_EDGE('',*,*,#14160,.F.);
#18615=ORIENTED_EDGE('',*,*,#14163,.T.);
#18616=ORIENTED_EDGE('',*,*,#14165,.F.);
#18617=ORIENTED_EDGE('',*,*,#14167,.T.);
#25481=CONICAL_SURFACE('',#27377,1.65,0.785398163397459);
#25482=CONICAL_SURFACE('',#27384,1.55,1.02974425867665);
#25483=CONICAL_SURFACE('',#27388,3.105,0.785398163397459);
#25484=CONICAL_SURFACE('',#27394,5.35,0.785398163397445);
#25716=ADVANCED_FACE('',(#2523),#2173,.T.);
#25717=ADVANCED_FACE('',(#2524),#1227,.F.);
#25718=ADVANCED_FACE('',(#2525),#2174,.F.);
#25719=ADVANCED_FACE('',(#2526),#2175,.F.);
#25720=ADVANCED_FACE('',(#2527),#2176,.F.);
#25721=ADVANCED_FACE('',(#2528),#2177,.F.);
#25722=ADVANCED_FACE('',(#2529),#25481,.F.);
#25723=ADVANCED_FACE('',(#2530),#2178,.F.);
#25724=ADVANCED_FACE('',(#2531,#1001),#1228,.T.);
#25725=ADVANCED_FACE('',(#2532),#25482,.F.);
#25726=ADVANCED_FACE('',(#2533),#2179,.T.);
#25727=ADVANCED_FACE('',(#2534),#25483,.T.);
#25728=ADVANCED_FACE('',(#2535),#2180,.T.);
#25729=ADVANCED_FACE('',(#2536,#1002),#1229,.T.);
#25730=ADVANCED_FACE('',(#2537),#25484,.T.);
#25731=ADVANCED_FACE('',(#2538),#1230,.T.);
#25732=ADVANCED_FACE('',(#2539),#2181,.T.);
#25733=ADVANCED_FACE('',(#2540),#2182,.T.);
#25734=ADVANCED_FACE('',(#2541),#1231,.T.);
#25735=ADVANCED_FACE('',(#2542),#2183,.T.);
#25736=ADVANCED_FACE('',(#2543),#2184,.T.);
#25737=ADVANCED_FACE('',(#2544,#1003),#1232,.T.);
#25738=ADVANCED_FACE('',(#2545,#1004,#1005),#1233,.T.);
#25739=ADVANCED_FACE('',(#2546,#1006,#1007),#1234,.T.);
#25740=ADVANCED_FACE('',(#2547,#1008,#1009),#1235,.F.);
#25741=ADVANCED_FACE('',(#2548),#1236,.T.);
#25742=ADVANCED_FACE('',(#2549),#2185,.T.);
#25743=ADVANCED_FACE('',(#2550),#1237,.T.);
#25744=ADVANCED_FACE('',(#2551),#2186,.T.);
#25745=ADVANCED_FACE('',(#2552),#1238,.T.);
#25746=ADVANCED_FACE('',(#2553),#2187,.T.);
#25747=ADVANCED_FACE('',(#2554),#1239,.T.);
#25748=ADVANCED_FACE('',(#2555),#2188,.T.);
#25749=ADVANCED_FACE('',(#2556,#1010,#1011),#1240,.F.);
#25750=ADVANCED_FACE('',(#2557),#1241,.T.);
#25751=ADVANCED_FACE('',(#2558),#1242,.T.);
#25752=ADVANCED_FACE('',(#2559),#2189,.T.);
#25753=ADVANCED_FACE('',(#2560),#1243,.T.);
#25754=ADVANCED_FACE('',(#2561),#2190,.T.);
#25755=ADVANCED_FACE('',(#2562,#1012),#1244,.T.);
#25756=ADVANCED_FACE('',(#2563),#2191,.T.);
#25757=ADVANCED_FACE('',(#2564),#1245,.T.);
#25758=ADVANCED_FACE('',(#2565),#2192,.T.);
#25759=ADVANCED_FACE('',(#2566),#1246,.T.);
#25760=ADVANCED_FACE('',(#2567),#1247,.F.);
#26931=CLOSED_SHELL('',(#25716,#25717,#25718,#25719,#25720,#25721,#25722,
#25723,#25724,#25725,#25726,#25727,#25728,#25729,#25730,#25731,#25732,#25733,
#25734,#25735,#25736,#25737,#25738,#25739,#25740,#25741,#25742,#25743,#25744,
#25745,#25746,#25747,#25748,#25749,#25750,#25751,#25752,#25753,#25754,#25755,
#25756,#25757,#25758,#25759,#25760));
#27360=AXIS2_PLACEMENT_3D('',#36901,#30091,#30092);
#27361=AXIS2_PLACEMENT_3D('',#36902,#30093,#30094);
#27362=AXIS2_PLACEMENT_3D('',#36904,#30095,#30096);
#27363=AXIS2_PLACEMENT_3D('',#36907,#30098,#30099);
#27364=AXIS2_PLACEMENT_3D('',#36908,#30100,#30101);
#27365=AXIS2_PLACEMENT_3D('',#36909,#30102,#30103);
#27366=AXIS2_PLACEMENT_3D('',#36911,#30104,#30105);
#27367=AXIS2_PLACEMENT_3D('',#36914,#30107,#30108);
#27368=AXIS2_PLACEMENT_3D('',#36915,#30109,#30110);
#27369=AXIS2_PLACEMENT_3D('',#36917,#30111,#30112);
#27370=AXIS2_PLACEMENT_3D('',#36920,#30114,#30115);
#27371=AXIS2_PLACEMENT_3D('',#36921,#30116,#30117);
#27372=AXIS2_PLACEMENT_3D('',#36923,#30118,#30119);
#27373=AXIS2_PLACEMENT_3D('',#36926,#30121,#30122);
#27374=AXIS2_PLACEMENT_3D('',#36927,#30123,#30124);
#27375=AXIS2_PLACEMENT_3D('',#36929,#30125,#30126);
#27376=AXIS2_PLACEMENT_3D('',#36932,#30128,#30129);
#27377=AXIS2_PLACEMENT_3D('',#36933,#30130,#30131);
#27378=AXIS2_PLACEMENT_3D('',#36935,#30132,#30133);
#27379=AXIS2_PLACEMENT_3D('',#36938,#30135,#30136);
#27380=AXIS2_PLACEMENT_3D('',#36939,#30137,#30138);
#27381=AXIS2_PLACEMENT_3D('',#36942,#30140,#30141);
#27382=AXIS2_PLACEMENT_3D('',#36943,#30142,#30143);
#27383=AXIS2_PLACEMENT_3D('',#36945,#30144,#30145);
#27384=AXIS2_PLACEMENT_3D('',#36946,#30146,#30147);
#27385=AXIS2_PLACEMENT_3D('',#36949,#30149,#30150);
#27386=AXIS2_PLACEMENT_3D('',#36951,#30151,#30152);
#27387=AXIS2_PLACEMENT_3D('',#36954,#30154,#30155);
#27388=AXIS2_PLACEMENT_3D('',#36955,#30156,#30157);
#27389=AXIS2_PLACEMENT_3D('',#36957,#30159,#30160);
#27390=AXIS2_PLACEMENT_3D('',#36959,#30161,#30162);
#27391=AXIS2_PLACEMENT_3D('',#36962,#30164,#30165);
#27392=AXIS2_PLACEMENT_3D('',#36963,#30166,#30167);
#27393=AXIS2_PLACEMENT_3D('',#36965,#30168,#30169);
#27394=AXIS2_PLACEMENT_3D('',#36966,#30170,#30171);
#27395=AXIS2_PLACEMENT_3D('',#36968,#30173,#30174);
#27396=AXIS2_PLACEMENT_3D('',#36977,#30179,#30180);
#27397=AXIS2_PLACEMENT_3D('',#36979,#30181,#30182);
#27398=AXIS2_PLACEMENT_3D('',#36981,#30183,#30184);
#27399=AXIS2_PLACEMENT_3D('',#36983,#30186,#30187);
#27400=AXIS2_PLACEMENT_3D('',#36986,#30188,#30189);
#27401=AXIS2_PLACEMENT_3D('',#36990,#30191,#30192);
#27402=AXIS2_PLACEMENT_3D('',#36992,#30194,#30195);
#27403=AXIS2_PLACEMENT_3D('',#36998,#30199,#30200);
#27404=AXIS2_PLACEMENT_3D('',#37000,#30201,#30202);
#27405=AXIS2_PLACEMENT_3D('',#37002,#30203,#30204);
#27406=AXIS2_PLACEMENT_3D('',#37004,#30206,#30207);
#27407=AXIS2_PLACEMENT_3D('',#37006,#30208,#30209);
#27408=AXIS2_PLACEMENT_3D('',#37009,#30211,#30212);
#27409=AXIS2_PLACEMENT_3D('',#37010,#30213,#30214);
#27410=AXIS2_PLACEMENT_3D('',#37013,#30217,#30218);
#27411=AXIS2_PLACEMENT_3D('',#37017,#30220,#30221);
#27412=AXIS2_PLACEMENT_3D('',#37021,#30223,#30224);
#27413=AXIS2_PLACEMENT_3D('',#37023,#30226,#30227);
#27414=AXIS2_PLACEMENT_3D('',#37027,#30229,#30230);
#27415=AXIS2_PLACEMENT_3D('',#37031,#30232,#30233);
#27416=AXIS2_PLACEMENT_3D('',#37033,#30235,#30236);
#27417=AXIS2_PLACEMENT_3D('',#37036,#30237,#30238);
#27418=AXIS2_PLACEMENT_3D('',#37040,#30240,#30241);
#27419=AXIS2_PLACEMENT_3D('',#37044,#30243,#30244);
#27420=AXIS2_PLACEMENT_3D('',#37048,#30246,#30247);
#27421=AXIS2_PLACEMENT_3D('',#37050,#30249,#30250);
#27422=AXIS2_PLACEMENT_3D('',#37053,#30253,#30254);
#27423=AXIS2_PLACEMENT_3D('',#37055,#30256,#30257);
#27424=AXIS2_PLACEMENT_3D('',#37061,#30261,#30262);
#27425=AXIS2_PLACEMENT_3D('',#37063,#30263,#30264);
#27426=AXIS2_PLACEMENT_3D('',#37065,#30266,#30267);
#27427=AXIS2_PLACEMENT_3D('',#37069,#30270,#30271);
#27428=AXIS2_PLACEMENT_3D('',#37071,#30272,#30273);
#27429=AXIS2_PLACEMENT_3D('',#37073,#30275,#30276);
#27430=AXIS2_PLACEMENT_3D('',#37078,#30280,#30281);
#27431=AXIS2_PLACEMENT_3D('',#37079,#30282,#30283);
#27432=AXIS2_PLACEMENT_3D('',#37081,#30284,#30285);
#27433=AXIS2_PLACEMENT_3D('',#37083,#30286,#30287);
#27434=AXIS2_PLACEMENT_3D('',#37085,#30289,#30290);
#27435=AXIS2_PLACEMENT_3D('',#37087,#30291,#30292);
#27436=AXIS2_PLACEMENT_3D('',#37090,#30294,#30295);
#27437=AXIS2_PLACEMENT_3D('',#37091,#30296,#30297);
#27438=AXIS2_PLACEMENT_3D('',#37097,#30301,#30302);
#27439=AXIS2_PLACEMENT_3D('',#37099,#30303,#30304);
#27440=AXIS2_PLACEMENT_3D('',#37101,#30305,#30306);
#27441=AXIS2_PLACEMENT_3D('',#37103,#30308,#30309);
#27442=AXIS2_PLACEMENT_3D('',#37109,#30313,#30314);
#27443=AXIS2_PLACEMENT_3D('',#37111,#30315,#30316);
#27444=AXIS2_PLACEMENT_3D('',#37112,#30317,#30318);
#27445=AXIS2_PLACEMENT_3D('',#37114,#30320,#30321);
#27446=AXIS2_PLACEMENT_3D('',#37118,#30324,#30325);
#27447=AXIS2_PLACEMENT_3D('',#37120,#30326,#30327);
#27448=AXIS2_PLACEMENT_3D('',#37122,#30329,#30330);
#27449=AXIS2_PLACEMENT_3D('',#37126,#30333,#30334);
#27450=AXIS2_PLACEMENT_3D('',#37127,#30335,#30336);
#27451=AXIS2_PLACEMENT_3D('',#37128,#30337,#30338);
#27452=AXIS2_PLACEMENT_3D('',#37129,#30339,#30340);
#30091=DIRECTION('axis',(0.,0.,1.));
#30092=DIRECTION('refdir',(1.,0.,0.));
#30093=DIRECTION('center_axis',(-1.,0.,0.));
#30094=DIRECTION('ref_axis',(0.,0.,-1.));
#30095=DIRECTION('center_axis',(-1.,0.,0.));
#30096=DIRECTION('ref_axis',(0.,0.,-1.));
#30097=DIRECTION('',(1.,0.,0.));
#30098=DIRECTION('center_axis',(1.,0.,0.));
#30099=DIRECTION('ref_axis',(0.,0.,-1.));
#30100=DIRECTION('center_axis',(1.,0.,0.));
#30101=DIRECTION('ref_axis',(0.,0.,-1.));
#30102=DIRECTION('center_axis',(0.,-1.,0.));
#30103=DIRECTION('ref_axis',(1.,0.,0.));
#30104=DIRECTION('center_axis',(0.,-1.,0.));
#30105=DIRECTION('ref_axis',(1.,0.,0.));
#30106=DIRECTION('',(0.,-1.,0.));
#30107=DIRECTION('center_axis',(0.,1.,0.));
#30108=DIRECTION('ref_axis',(1.,0.,0.));
#30109=DIRECTION('center_axis',(0.,-1.,0.));
#30110=DIRECTION('ref_axis',(1.,0.,0.));
#30111=DIRECTION('center_axis',(0.,-1.,0.));
#30112=DIRECTION('ref_axis',(1.,0.,0.));
#30113=DIRECTION('',(0.,-1.,0.));
#30114=DIRECTION('center_axis',(0.,1.,0.));
#30115=DIRECTION('ref_axis',(1.,0.,0.));
#30116=DIRECTION('center_axis',(0.,-1.,0.));
#30117=DIRECTION('ref_axis',(1.,0.,0.));
#30118=DIRECTION('center_axis',(0.,-1.,0.));
#30119=DIRECTION('ref_axis',(1.,0.,0.));
#30120=DIRECTION('',(0.,-1.,0.));
#30121=DIRECTION('center_axis',(0.,1.,0.));
#30122=DIRECTION('ref_axis',(1.,0.,0.));
#30123=DIRECTION('center_axis',(0.,-1.,0.));
#30124=DIRECTION('ref_axis',(1.,0.,0.));
#30125=DIRECTION('center_axis',(0.,-1.,0.));
#30126=DIRECTION('ref_axis',(1.,0.,0.));
#30127=DIRECTION('',(0.,-1.,0.));
#30128=DIRECTION('center_axis',(0.,1.,0.));
#30129=DIRECTION('ref_axis',(1.,0.,0.));
#30130=DIRECTION('center_axis',(0.,1.,0.));
#30131=DIRECTION('ref_axis',(1.,0.,0.));
#30132=DIRECTION('center_axis',(0.,-1.,0.));
#30133=DIRECTION('ref_axis',(1.,0.,0.));
#30134=DIRECTION('',(-0.707106781186555,0.70710678118654,8.65956056235503E-17));
#30135=DIRECTION('center_axis',(0.,1.,0.));
#30136=DIRECTION('ref_axis',(1.,0.,0.));
#30137=DIRECTION('center_axis',(0.,-1.,0.));
#30138=DIRECTION('ref_axis',(1.,0.,0.));
#30139=DIRECTION('',(0.,-1.,0.));
#30140=DIRECTION('center_axis',(0.,-1.,0.));
#30141=DIRECTION('ref_axis',(1.,0.,0.));
#30142=DIRECTION('center_axis',(0.,1.,0.));
#30143=DIRECTION('ref_axis',(0.,0.,1.));
#30144=DIRECTION('center_axis',(0.,-1.,0.));
#30145=DIRECTION('ref_axis',(1.,0.,0.));
#30146=DIRECTION('center_axis',(0.,1.,0.));
#30147=DIRECTION('ref_axis',(1.,0.,0.));
#30148=DIRECTION('',(-0.85716730070211,0.515038074910058,1.04972719113862E-16));
#30149=DIRECTION('center_axis',(0.,-1.,0.));
#30150=DIRECTION('ref_axis',(1.,0.,0.));
#30151=DIRECTION('center_axis',(0.,-1.,0.));
#30152=DIRECTION('ref_axis',(1.,0.,0.));
#30153=DIRECTION('',(0.,1.,0.));
#30154=DIRECTION('center_axis',(0.,-1.,0.));
#30155=DIRECTION('ref_axis',(1.,0.,0.));
#30156=DIRECTION('center_axis',(0.,-1.,0.));
#30157=DIRECTION('ref_axis',(1.,0.,0.));
#30158=DIRECTION('',(0.707106781186555,0.70710678118654,8.65956056235503E-17));
#30159=DIRECTION('center_axis',(0.,-1.,0.));
#30160=DIRECTION('ref_axis',(1.,0.,0.));
#30161=DIRECTION('center_axis',(0.,-1.,0.));
#30162=DIRECTION('ref_axis',(1.,0.,0.));
#30163=DIRECTION('',(0.,1.,0.));
#30164=DIRECTION('center_axis',(0.,-1.,0.));
#30165=DIRECTION('ref_axis',(1.,0.,0.));
#30166=DIRECTION('center_axis',(0.,1.,0.));
#30167=DIRECTION('ref_axis',(0.,0.,1.));
#30168=DIRECTION('center_axis',(0.,-1.,0.));
#30169=DIRECTION('ref_axis',(1.,0.,0.));
#30170=DIRECTION('center_axis',(0.,-1.,0.));
#30171=DIRECTION('ref_axis',(1.,0.,0.));
#30172=DIRECTION('',(0.707106781186545,0.70710678118655,8.6595605623549E-17));
#30173=DIRECTION('center_axis',(1.,0.,0.));
#30174=DIRECTION('ref_axis',(0.,0.,-1.));
#30175=DIRECTION('',(0.,0.,1.));
#30176=DIRECTION('',(0.,1.,0.));
#30177=DIRECTION('',(0.,0.,-1.));
#30178=DIRECTION('',(0.,1.,0.));
#30179=DIRECTION('center_axis',(0.,1.,0.));
#30180=DIRECTION('ref_axis',(0.,0.,1.));
#30181=DIRECTION('center_axis',(0.,-1.,0.));
#30182=DIRECTION('ref_axis',(0.,0.,1.));
#30183=DIRECTION('center_axis',(0.,1.,0.));
#30184=DIRECTION('ref_axis',(0.,0.,1.));
#30185=DIRECTION('',(0.,1.,0.));
#30186=DIRECTION('center_axis',(0.,1.,0.));
#30187=DIRECTION('ref_axis',(-1.,0.,1.48029736616687E-15));
#30188=DIRECTION('center_axis',(0.,-1.,0.));
#30189=DIRECTION('ref_axis',(-1.,0.,1.48029736616687E-15));
#30190=DIRECTION('',(0.,1.,0.));
#30191=DIRECTION('center_axis',(0.,1.,0.));
#30192=DIRECTION('ref_axis',(-1.,0.,1.48029736616687E-15));
#30193=DIRECTION('',(0.,1.,0.));
#30194=DIRECTION('center_axis',(-1.,0.,0.));
#30195=DIRECTION('ref_axis',(0.,0.,1.));
#30196=DIRECTION('',(0.,0.,-1.));
#30197=DIRECTION('',(0.,0.,1.));
#30198=DIRECTION('',(0.,1.,0.));
#30199=DIRECTION('center_axis',(0.,1.,0.));
#30200=DIRECTION('ref_axis',(-1.48029736616687E-15,0.,-1.));
#30201=DIRECTION('center_axis',(0.,-1.,0.));
#30202=DIRECTION('ref_axis',(-1.48029736616687E-15,0.,-1.));
#30203=DIRECTION('center_axis',(0.,1.,0.));
#30204=DIRECTION('ref_axis',(-1.48029736616687E-15,0.,-1.));
#30205=DIRECTION('',(0.,1.,0.));
#30206=DIRECTION('center_axis',(0.,1.,0.));
#30207=DIRECTION('ref_axis',(1.,0.,1.48029736616688E-15));
#30208=DIRECTION('center_axis',(0.,-1.,0.));
#30209=DIRECTION('ref_axis',(1.,0.,1.48029736616688E-15));
#30210=DIRECTION('',(0.,1.,0.));
#30211=DIRECTION('center_axis',(0.,1.,0.));
#30212=DIRECTION('ref_axis',(1.,0.,1.48029736616688E-15));
#30213=DIRECTION('center_axis',(0.,1.,0.));
#30214=DIRECTION('ref_axis',(1.,0.,0.));
#30215=DIRECTION('',(-1.,0.,0.));
#30216=DIRECTION('',(1.,0.,0.));
#30217=DIRECTION('center_axis',(0.,1.,0.));
#30218=DIRECTION('ref_axis',(1.,0.,0.));
#30219=DIRECTION('',(1.,0.,0.));
#30220=DIRECTION('center_axis',(0.,1.,0.));
#30221=DIRECTION('ref_axis',(-8.88178419700132E-15,0.,1.));
#30222=DIRECTION('',(0.,0.,-1.));
#30223=DIRECTION('center_axis',(0.,1.,0.));
#30224=DIRECTION('ref_axis',(1.,0.,6.66133814775096E-15));
#30225=DIRECTION('',(-1.,0.,0.));
#30226=DIRECTION('center_axis',(0.,1.,0.));
#30227=DIRECTION('ref_axis',(1.,0.,0.));
#30228=DIRECTION('',(-1.,0.,0.));
#30229=DIRECTION('center_axis',(0.,1.,0.));
#30230=DIRECTION('ref_axis',(0.,0.,-1.));
#30231=DIRECTION('',(0.,0.,1.));
#30232=DIRECTION('center_axis',(0.,1.,0.));
#30233=DIRECTION('ref_axis',(-1.,0.,0.));
#30234=DIRECTION('',(1.,0.,0.));
#30235=DIRECTION('center_axis',(0.,1.,0.));
#30236=DIRECTION('ref_axis',(1.,0.,0.));
#30237=DIRECTION('center_axis',(0.,1.,0.));
#30238=DIRECTION('ref_axis',(0.,0.,1.));
#30239=DIRECTION('',(0.,0.,-1.));
#30240=DIRECTION('center_axis',(0.,1.,0.));
#30241=DIRECTION('ref_axis',(1.,0.,1.48029736616688E-15));
#30242=DIRECTION('',(1.,0.,0.));
#30243=DIRECTION('center_axis',(0.,1.,0.));
#30244=DIRECTION('ref_axis',(1.,0.,6.66133814775096E-15));
#30245=DIRECTION('',(0.,0.,1.));
#30246=DIRECTION('center_axis',(0.,1.,0.));
#30247=DIRECTION('ref_axis',(-8.88178419700132E-15,0.,1.));
#30248=DIRECTION('',(-1.,0.,0.));
#30249=DIRECTION('center_axis',(1.,0.,0.));
#30250=DIRECTION('ref_axis',(0.,0.,-1.));
#30251=DIRECTION('',(0.,1.,0.));
#30252=DIRECTION('',(0.,1.,0.));
#30253=DIRECTION('center_axis',(0.,1.,0.));
#30254=DIRECTION('ref_axis',(-8.88178419700132E-15,0.,1.));
#30255=DIRECTION('',(0.,1.,0.));
#30256=DIRECTION('center_axis',(0.,0.,1.));
#30257=DIRECTION('ref_axis',(1.,0.,0.));
#30258=DIRECTION('',(0.,1.,0.));
#30259=DIRECTION('',(-1.,0.,0.));
#30260=DIRECTION('',(-1.,0.,0.));
#30261=DIRECTION('center_axis',(0.,1.,0.));
#30262=DIRECTION('ref_axis',(-1.,0.,0.));
#30263=DIRECTION('center_axis',(0.,1.,0.));
#30264=DIRECTION('ref_axis',(-1.,0.,0.));
#30265=DIRECTION('',(0.,1.,0.));
#30266=DIRECTION('center_axis',(-1.,0.,0.));
#30267=DIRECTION('ref_axis',(0.,0.,1.));
#30268=DIRECTION('',(0.,0.,-1.));
#30269=DIRECTION('',(0.,1.,0.));
#30270=DIRECTION('center_axis',(0.,1.,0.));
#30271=DIRECTION('ref_axis',(0.,0.,-1.));
#30272=DIRECTION('center_axis',(0.,1.,0.));
#30273=DIRECTION('ref_axis',(0.,0.,-1.));
#30274=DIRECTION('',(0.,1.,0.));
#30275=DIRECTION('center_axis',(0.,0.,-1.));
#30276=DIRECTION('ref_axis',(-1.,0.,0.));
#30277=DIRECTION('',(1.,0.,0.));
#30278=DIRECTION('',(0.,1.,0.));
#30279=DIRECTION('',(1.,0.,0.));
#30280=DIRECTION('center_axis',(0.,1.,0.));
#30281=DIRECTION('ref_axis',(1.,0.,6.66133814775096E-15));
#30282=DIRECTION('center_axis',(0.,1.,0.));
#30283=DIRECTION('ref_axis',(1.,0.,0.));
#30284=DIRECTION('center_axis',(0.,1.,0.));
#30285=DIRECTION('ref_axis',(-1.,0.,1.48029736616688E-15));
#30286=DIRECTION('center_axis',(0.,1.,0.));
#30287=DIRECTION('ref_axis',(1.48029736616687E-15,0.,-1.));
#30288=DIRECTION('',(0.,0.,1.));
#30289=DIRECTION('center_axis',(0.,1.,0.));
#30290=DIRECTION('ref_axis',(1.,0.,0.));
#30291=DIRECTION('center_axis',(0.,1.,0.));
#30292=DIRECTION('ref_axis',(1.,0.,1.48029736616688E-15));
#30293=DIRECTION('',(-1.,0.,0.));
#30294=DIRECTION('center_axis',(0.,1.,0.));
#30295=DIRECTION('ref_axis',(1.48029736616687E-15,0.,-1.));
#30296=DIRECTION('center_axis',(1.,0.,0.));
#30297=DIRECTION('ref_axis',(0.,0.,-1.));
#30298=DIRECTION('',(0.,0.,1.));
#30299=DIRECTION('',(0.,1.,0.));
#30300=DIRECTION('',(0.,1.,0.));
#30301=DIRECTION('center_axis',(0.,1.,0.));
#30302=DIRECTION('ref_axis',(0.,0.,1.));
#30303=DIRECTION('center_axis',(0.,1.,0.));
#30304=DIRECTION('ref_axis',(0.,0.,1.));
#30305=DIRECTION('center_axis',(0.,1.,0.));
#30306=DIRECTION('ref_axis',(0.,0.,1.));
#30307=DIRECTION('',(0.,1.,0.));
#30308=DIRECTION('center_axis',(0.,0.,1.));
#30309=DIRECTION('ref_axis',(1.,0.,0.));
#30310=DIRECTION('',(-1.,0.,0.));
#30311=DIRECTION('',(1.,0.,0.));
#30312=DIRECTION('',(0.,1.,0.));
#30313=DIRECTION('center_axis',(0.,1.,0.));
#30314=DIRECTION('ref_axis',(-1.,0.,1.48029736616688E-15));
#30315=DIRECTION('center_axis',(0.,1.,0.));
#30316=DIRECTION('ref_axis',(-1.,0.,1.48029736616688E-15));
#30317=DIRECTION('center_axis',(0.,1.,0.));
#30318=DIRECTION('ref_axis',(-1.,0.,1.48029736616688E-15));
#30319=DIRECTION('',(0.,1.,0.));
#30320=DIRECTION('center_axis',(-1.,0.,0.));
#30321=DIRECTION('ref_axis',(0.,0.,1.));
#30322=DIRECTION('',(0.,0.,-1.));
#30323=DIRECTION('',(0.,1.,0.));
#30324=DIRECTION('center_axis',(0.,1.,0.));
#30325=DIRECTION('ref_axis',(1.48029736616687E-15,0.,-1.));
#30326=DIRECTION('center_axis',(0.,1.,0.));
#30327=DIRECTION('ref_axis',(1.48029736616687E-15,0.,-1.));
#30328=DIRECTION('',(0.,1.,0.));
#30329=DIRECTION('center_axis',(0.,0.,-1.));
#30330=DIRECTION('ref_axis',(-1.,0.,0.));
#30331=DIRECTION('',(1.,0.,0.));
#30332=DIRECTION('',(0.,1.,0.));
#30333=DIRECTION('center_axis',(0.,1.,0.));
#30334=DIRECTION('ref_axis',(1.,0.,1.48029736616688E-15));
#30335=DIRECTION('center_axis',(0.,1.,0.));
#30336=DIRECTION('ref_axis',(1.,0.,1.48029736616688E-15));
#30337=DIRECTION('center_axis',(0.,1.,0.));
#30338=DIRECTION('ref_axis',(1.,0.,0.));
#30339=DIRECTION('center_axis',(0.,1.,0.));
#30340=DIRECTION('ref_axis',(1.,0.,0.));
#36901=CARTESIAN_POINT('',(0.,0.,0.));
#36902=CARTESIAN_POINT('Origin',(-13.82,8.,0.));
#36903=CARTESIAN_POINT('',(-17.82,8.,2.5));
#36904=CARTESIAN_POINT('Origin',(-17.82,8.,0.));
#36905=CARTESIAN_POINT('',(-13.82,8.,2.5));
#36906=CARTESIAN_POINT('',(-13.82,8.,2.5));
#36907=CARTESIAN_POINT('Origin',(-13.82,8.,0.));
#36908=CARTESIAN_POINT('Origin',(-17.82,8.,0.));
#36909=CARTESIAN_POINT('Origin',(49.34,41.616,-7.87));
#36910=CARTESIAN_POINT('',(47.34,41.616,-7.87));
#36911=CARTESIAN_POINT('Origin',(49.34,41.616,-7.87));
#36912=CARTESIAN_POINT('',(47.34,39.116,-7.87));
#36913=CARTESIAN_POINT('',(47.34,41.616,-7.87));
#36914=CARTESIAN_POINT('Origin',(49.34,39.116,-7.87));
#36915=CARTESIAN_POINT('Origin',(-17.98,41.616,7.87));
#36916=CARTESIAN_POINT('',(-19.98,41.616,7.87));
#36917=CARTESIAN_POINT('Origin',(-17.98,41.616,7.87));
#36918=CARTESIAN_POINT('',(-19.98,39.116,7.87));
#36919=CARTESIAN_POINT('',(-19.98,41.616,7.87));
#36920=CARTESIAN_POINT('Origin',(-17.98,39.116,7.87));
#36921=CARTESIAN_POINT('Origin',(-17.98,41.616,-7.87));
#36922=CARTESIAN_POINT('',(-19.98,41.616,-7.87));
#36923=CARTESIAN_POINT('Origin',(-17.98,41.616,-7.87));
#36924=CARTESIAN_POINT('',(-19.98,39.116,-7.87));
#36925=CARTESIAN_POINT('',(-19.98,41.616,-7.87));
#36926=CARTESIAN_POINT('Origin',(-17.98,39.116,-7.87));
#36927=CARTESIAN_POINT('Origin',(49.34,41.616,7.87));
#36928=CARTESIAN_POINT('',(47.34,41.616,7.87));
#36929=CARTESIAN_POINT('Origin',(49.34,41.616,7.87));
#36930=CARTESIAN_POINT('',(47.34,39.116,7.87));
#36931=CARTESIAN_POINT('',(47.34,41.616,7.87));
#36932=CARTESIAN_POINT('Origin',(49.34,39.116,7.87));
#36933=CARTESIAN_POINT('Origin',(0.,53.835,0.));
#36934=CARTESIAN_POINT('',(-1.55,53.735,-1.8982025386784E-16));
#36935=CARTESIAN_POINT('Origin',(0.,53.735,0.));
#36936=CARTESIAN_POINT('',(-1.75,53.935,2.14313189850787E-16));
#36937=CARTESIAN_POINT('',(-1.65,53.835,2.02066721859313E-16));
#36938=CARTESIAN_POINT('Origin',(0.,53.935,0.));
#36939=CARTESIAN_POINT('Origin',(0.,53.935,0.));
#36940=CARTESIAN_POINT('',(-1.55,47.935,-1.8982025386784E-16));
#36941=CARTESIAN_POINT('',(-1.55,53.935,-1.8982025386784E-16));
#36942=CARTESIAN_POINT('Origin',(0.,47.935,0.));
#36943=CARTESIAN_POINT('Origin',(2.955,53.935,0.));
#36944=CARTESIAN_POINT('',(-2.955,53.935,-3.61883129148043E-16));
#36945=CARTESIAN_POINT('Origin',(0.,53.935,0.));
#36946=CARTESIAN_POINT('Origin',(0.,47.935,0.));
#36947=CARTESIAN_POINT('',(0.,47.0036660405073,0.));
#36948=CARTESIAN_POINT('',(-1.55,47.935,1.8982025386784E-16));
#36949=CARTESIAN_POINT('Origin',(0.,51.0675,0.));
#36950=CARTESIAN_POINT('',(-3.255,49.,-3.98622533122464E-16));
#36951=CARTESIAN_POINT('Origin',(0.,49.,0.));
#36952=CARTESIAN_POINT('',(-3.255,53.635,-3.98622533122464E-16));
#36953=CARTESIAN_POINT('',(-3.255,51.0675,-3.98622533122464E-16));
#36954=CARTESIAN_POINT('Origin',(0.,53.635,0.));
#36955=CARTESIAN_POINT('Origin',(0.,53.785,0.));
#36956=CARTESIAN_POINT('',(-3.105,53.785,-3.80252831135253E-16));
#36957=CARTESIAN_POINT('Origin',(0.,47.6,0.));
#36958=CARTESIAN_POINT('',(-5.5,47.,-6.73555739531044E-16));
#36959=CARTESIAN_POINT('Origin',(0.,47.,0.));
#36960=CARTESIAN_POINT('',(-5.5,48.7,-6.73555739531044E-16));
#36961=CARTESIAN_POINT('',(-5.5,47.6,-6.73555739531044E-16));
#36962=CARTESIAN_POINT('Origin',(0.,48.7,0.));
#36963=CARTESIAN_POINT('Origin',(5.2,49.,0.));
#36964=CARTESIAN_POINT('',(-5.2,49.,-6.36816335556623E-16));
#36965=CARTESIAN_POINT('Origin',(0.,49.,0.));
#36966=CARTESIAN_POINT('Origin',(0.,48.85,0.));
#36967=CARTESIAN_POINT('',(-5.35,48.85,-6.55186037543834E-16));
#36968=CARTESIAN_POINT('Origin',(44.98,41.616,12.5));
#36969=CARTESIAN_POINT('',(44.98,41.616,-12.5));
#36970=CARTESIAN_POINT('',(44.98,41.616,12.5));
#36971=CARTESIAN_POINT('',(44.98,41.616,6.25));
#36972=CARTESIAN_POINT('',(44.98,47.,-12.5));
#36973=CARTESIAN_POINT('',(44.98,41.616,-12.5));
#36974=CARTESIAN_POINT('',(44.98,47.,12.5));
#36975=CARTESIAN_POINT('',(44.98,47.,-12.5));
#36976=CARTESIAN_POINT('',(44.98,41.616,12.5));
#36977=CARTESIAN_POINT('Origin',(43.48,41.616,12.5));
#36978=CARTESIAN_POINT('',(43.48,41.616,14.));
#36979=CARTESIAN_POINT('Origin',(43.48,41.616,12.5));
#36980=CARTESIAN_POINT('',(43.48,47.,14.));
#36981=CARTESIAN_POINT('Origin',(43.48,47.,12.5));
#36982=CARTESIAN_POINT('',(43.48,41.616,14.));
#36983=CARTESIAN_POINT('Origin',(-12.12,41.616,12.5));
#36984=CARTESIAN_POINT('',(-12.12,41.616,14.));
#36985=CARTESIAN_POINT('',(-13.62,41.616,12.5));
#36986=CARTESIAN_POINT('Origin',(-12.12,41.616,12.5));
#36987=CARTESIAN_POINT('',(-12.12,47.,14.));
#36988=CARTESIAN_POINT('',(-12.12,41.616,14.));
#36989=CARTESIAN_POINT('',(-13.62,47.,12.5));
#36990=CARTESIAN_POINT('Origin',(-12.12,47.,12.5));
#36991=CARTESIAN_POINT('',(-13.62,41.616,12.5));
#36992=CARTESIAN_POINT('Origin',(-13.62,41.616,-12.5));
#36993=CARTESIAN_POINT('',(-13.62,41.616,-12.5));
#36994=CARTESIAN_POINT('',(-13.62,41.616,-6.25));
#36995=CARTESIAN_POINT('',(-13.62,47.,-12.5));
#36996=CARTESIAN_POINT('',(-13.62,47.,12.5));
#36997=CARTESIAN_POINT('',(-13.62,41.616,-12.5));
#36998=CARTESIAN_POINT('Origin',(-12.12,41.616,-12.5));
#36999=CARTESIAN_POINT('',(-12.12,41.616,-14.));
#37000=CARTESIAN_POINT('Origin',(-12.12,41.616,-12.5));
#37001=CARTESIAN_POINT('',(-12.12,47.,-14.));
#37002=CARTESIAN_POINT('Origin',(-12.12,47.,-12.5));
#37003=CARTESIAN_POINT('',(-12.12,41.616,-14.));
#37004=CARTESIAN_POINT('Origin',(43.48,41.616,-12.5));
#37005=CARTESIAN_POINT('',(43.48,41.616,-14.));
#37006=CARTESIAN_POINT('Origin',(43.48,41.616,-12.5));
#37007=CARTESIAN_POINT('',(43.48,47.,-14.));
#37008=CARTESIAN_POINT('',(43.48,41.616,-14.));
#37009=CARTESIAN_POINT('Origin',(43.48,47.,-12.5));
#37010=CARTESIAN_POINT('Origin',(15.68,47.,0.));
#37011=CARTESIAN_POINT('',(-12.12,47.,-14.));
#37012=CARTESIAN_POINT('',(43.48,47.,14.));
#37013=CARTESIAN_POINT('Origin',(15.68,41.616,-2.22044604925031E-15));
#37014=CARTESIAN_POINT('',(51.68,41.616,14.));
#37015=CARTESIAN_POINT('',(51.68,41.616,14.));
#37016=CARTESIAN_POINT('',(52.68,41.616,13.));
#37017=CARTESIAN_POINT('Origin',(51.68,41.616,13.));
#37018=CARTESIAN_POINT('',(52.68,41.616,-13.));
#37019=CARTESIAN_POINT('',(52.68,41.616,-13.));
#37020=CARTESIAN_POINT('',(51.68,41.616,-14.));
#37021=CARTESIAN_POINT('Origin',(51.68,41.616,-13.));
#37022=CARTESIAN_POINT('',(-20.32,41.616,-14.));
#37023=CARTESIAN_POINT('Origin',(15.68,41.616,-2.22044604925031E-15));
#37024=CARTESIAN_POINT('',(-20.32,41.616,-14.));
#37025=CARTESIAN_POINT('',(-20.32,41.616,-14.));
#37026=CARTESIAN_POINT('',(-21.32,41.616,-13.));
#37027=CARTESIAN_POINT('Origin',(-20.32,41.616,-13.));
#37028=CARTESIAN_POINT('',(-21.32,41.616,13.));
#37029=CARTESIAN_POINT('',(-21.32,41.616,13.));
#37030=CARTESIAN_POINT('',(-20.32,41.616,14.));
#37031=CARTESIAN_POINT('Origin',(-20.32,41.616,13.));
#37032=CARTESIAN_POINT('',(51.68,41.616,14.));
#37033=CARTESIAN_POINT('Origin',(15.68,39.116,-2.22044604925031E-15));
#37034=CARTESIAN_POINT('',(44.6998039027186,39.116,14.));
#37035=CARTESIAN_POINT('',(45.18,39.116,12.9));
#37036=CARTESIAN_POINT('Origin',(43.68,39.116,12.9));
#37037=CARTESIAN_POINT('',(45.18,39.116,-12.9));
#37038=CARTESIAN_POINT('',(45.18,39.116,-12.9));
#37039=CARTESIAN_POINT('',(44.6998039027186,39.116,-14.));
#37040=CARTESIAN_POINT('Origin',(43.68,39.116,-12.9));
#37041=CARTESIAN_POINT('',(51.68,39.116,-14.));
#37042=CARTESIAN_POINT('',(-20.32,39.116,-14.));
#37043=CARTESIAN_POINT('',(52.68,39.116,-13.));
#37044=CARTESIAN_POINT('Origin',(51.68,39.116,-13.));
#37045=CARTESIAN_POINT('',(52.68,39.116,13.));
#37046=CARTESIAN_POINT('',(52.68,39.116,-13.));
#37047=CARTESIAN_POINT('',(51.68,39.116,14.));
#37048=CARTESIAN_POINT('Origin',(51.68,39.116,13.));
#37049=CARTESIAN_POINT('',(51.68,39.116,14.));
#37050=CARTESIAN_POINT('Origin',(52.68,39.116,13.));
#37051=CARTESIAN_POINT('',(52.68,39.116,-13.));
#37052=CARTESIAN_POINT('',(52.68,39.116,13.));
#37053=CARTESIAN_POINT('Origin',(51.68,39.116,13.));
#37054=CARTESIAN_POINT('',(51.68,39.116,14.));
#37055=CARTESIAN_POINT('Origin',(-20.32,39.116,14.));
#37056=CARTESIAN_POINT('',(-20.32,39.116,14.));
#37057=CARTESIAN_POINT('',(-20.32,39.116,14.));
#37058=CARTESIAN_POINT('',(-13.3398039027186,39.116,14.));
#37059=CARTESIAN_POINT('',(51.68,39.116,14.));
#37060=CARTESIAN_POINT('',(-2.32,39.116,14.));
#37061=CARTESIAN_POINT('Origin',(-20.32,39.116,13.));
#37062=CARTESIAN_POINT('',(-21.32,39.116,13.));
#37063=CARTESIAN_POINT('Origin',(-20.32,39.116,13.));
#37064=CARTESIAN_POINT('',(-21.32,39.116,13.));
#37065=CARTESIAN_POINT('Origin',(-21.32,39.116,-13.));
#37066=CARTESIAN_POINT('',(-21.32,39.116,-13.));
#37067=CARTESIAN_POINT('',(-21.32,39.116,13.));
#37068=CARTESIAN_POINT('',(-21.32,39.116,-13.));
#37069=CARTESIAN_POINT('Origin',(-20.32,39.116,-13.));
#37070=CARTESIAN_POINT('',(-20.32,39.116,-14.));
#37071=CARTESIAN_POINT('Origin',(-20.32,39.116,-13.));
#37072=CARTESIAN_POINT('',(-20.32,39.116,-14.));
#37073=CARTESIAN_POINT('Origin',(51.68,39.116,-14.));
#37074=CARTESIAN_POINT('',(-13.3398039027186,39.116,-14.));
#37075=CARTESIAN_POINT('',(-20.32,39.116,-14.));
#37076=CARTESIAN_POINT('',(51.68,39.116,-14.));
#37077=CARTESIAN_POINT('',(33.68,39.116,-14.));
#37078=CARTESIAN_POINT('Origin',(51.68,39.116,-13.));
#37079=CARTESIAN_POINT('Origin',(15.68,39.116,-2.22044604925031E-15));
#37080=CARTESIAN_POINT('',(-13.82,39.116,12.9));
#37081=CARTESIAN_POINT('Origin',(-12.32,39.116,12.9));
#37082=CARTESIAN_POINT('',(-13.82,39.116,-12.9));
#37083=CARTESIAN_POINT('Origin',(-12.32,39.116,-12.9));
#37084=CARTESIAN_POINT('',(-13.82,39.116,12.9));
#37085=CARTESIAN_POINT('Origin',(15.68,39.116,0.));
#37086=CARTESIAN_POINT('',(43.68,39.116,-14.4));
#37087=CARTESIAN_POINT('Origin',(43.68,39.116,-12.9));
#37088=CARTESIAN_POINT('',(-12.32,39.116,-14.4));
#37089=CARTESIAN_POINT('',(-12.32,39.116,-14.4));
#37090=CARTESIAN_POINT('Origin',(-12.32,39.116,-12.9));
#37091=CARTESIAN_POINT('Origin',(45.18,0.,12.9));
#37092=CARTESIAN_POINT('',(45.18,0.,-12.9));
#37093=CARTESIAN_POINT('',(45.18,0.,12.9));
#37094=CARTESIAN_POINT('',(45.18,0.,-12.9));
#37095=CARTESIAN_POINT('',(45.18,0.,-12.9));
#37096=CARTESIAN_POINT('',(45.18,0.,12.9));
#37097=CARTESIAN_POINT('Origin',(43.68,0.,12.9));
#37098=CARTESIAN_POINT('',(43.68,0.,14.4));
#37099=CARTESIAN_POINT('Origin',(43.68,0.,12.9));
#37100=CARTESIAN_POINT('',(43.68,39.116,14.4));
#37101=CARTESIAN_POINT('Origin',(43.68,39.116,12.9));
#37102=CARTESIAN_POINT('',(43.68,0.,14.4));
#37103=CARTESIAN_POINT('Origin',(-12.32,0.,14.4));
#37104=CARTESIAN_POINT('',(-12.32,0.,14.4));
#37105=CARTESIAN_POINT('',(43.68,0.,14.4));
#37106=CARTESIAN_POINT('',(-12.32,39.116,14.4));
#37107=CARTESIAN_POINT('',(43.68,39.116,14.4));
#37108=CARTESIAN_POINT('',(-12.32,0.,14.4));
#37109=CARTESIAN_POINT('Origin',(-12.32,0.,12.9));
#37110=CARTESIAN_POINT('',(-13.82,0.,12.9));
#37111=CARTESIAN_POINT('Origin',(-12.32,0.,12.9));
#37112=CARTESIAN_POINT('Origin',(-12.32,39.116,12.9));
#37113=CARTESIAN_POINT('',(-13.82,0.,12.9));
#37114=CARTESIAN_POINT('Origin',(-13.82,0.,-12.9));
#37115=CARTESIAN_POINT('',(-13.82,0.,-12.9));
#37116=CARTESIAN_POINT('',(-13.82,0.,12.9));
#37117=CARTESIAN_POINT('',(-13.82,0.,-12.9));
#37118=CARTESIAN_POINT('Origin',(-12.32,0.,-12.9));
#37119=CARTESIAN_POINT('',(-12.32,0.,-14.4));
#37120=CARTESIAN_POINT('Origin',(-12.32,0.,-12.9));
#37121=CARTESIAN_POINT('',(-12.32,0.,-14.4));
#37122=CARTESIAN_POINT('Origin',(43.68,0.,-14.4));
#37123=CARTESIAN_POINT('',(43.68,0.,-14.4));
#37124=CARTESIAN_POINT('',(-12.32,0.,-14.4));
#37125=CARTESIAN_POINT('',(43.68,0.,-14.4));
#37126=CARTESIAN_POINT('Origin',(43.68,0.,-12.9));
#37127=CARTESIAN_POINT('Origin',(43.68,0.,-12.9));
#37128=CARTESIAN_POINT('Origin',(15.68,39.116,0.));
#37129=CARTESIAN_POINT('Origin',(15.68,0.,0.));
#83191=UNCERTAINTY_MEASURE_WITH_UNIT(LENGTH_MEASURE(0.01),#83220,
'DISTANCE_ACCURACY_VALUE',
'Maximum model space distance between geometric entities at asserted c
onnectivities');
#83203=UNCERTAINTY_MEASURE_WITH_UNIT(LENGTH_MEASURE(0.01),#83220,
'DISTANCE_ACCURACY_VALUE',
'Maximum model space distance between geometric entities at asserted c
onnectivities');
#83207=(
GEOMETRIC_REPRESENTATION_CONTEXT(3)
GLOBAL_UNCERTAINTY_ASSIGNED_CONTEXT((#83191))
GLOBAL_UNIT_ASSIGNED_CONTEXT((#83220,#83222,#83223))
REPRESENTATION_CONTEXT('','3D')
);
#83219=(
GEOMETRIC_REPRESENTATION_CONTEXT(3)
GLOBAL_UNCERTAINTY_ASSIGNED_CONTEXT((#83203))
GLOBAL_UNIT_ASSIGNED_CONTEXT((#83220,#83222,#83223))
REPRESENTATION_CONTEXT('','3D')
);
#83220=(
LENGTH_UNIT()
NAMED_UNIT(*)
SI_UNIT(.MILLI.,.METRE.)
);
#83222=(
NAMED_UNIT(*)
PLANE_ANGLE_UNIT()
SI_UNIT($,.RADIAN.)
);
#83223=(
NAMED_UNIT(*)
SI_UNIT($,.STERADIAN.)
SOLID_ANGLE_UNIT()
);
#83227=SHAPE_DEFINITION_REPRESENTATION(#83242,#83302);
#83242=PRODUCT_DEFINITION_SHAPE('',$,#83318);
#83302=SHAPE_REPRESENTATION('',(#27360),#83207);
#83314=PRODUCT_DEFINITION_CONTEXT('part definition',#83361,'design');
#83318=PRODUCT_DEFINITION('Winch Servo','Winch Servo',#83333,#83314);
#83333=PRODUCT_DEFINITION_FORMATION('',$,#83366);
#83361=APPLICATION_CONTEXT(
'Core Data for Automotive Mechanical Design Process');
#83362=PRODUCT_CONTEXT('part definition',#83361,'mechanical');
#83366=PRODUCT('Winch Servo','Winch Servo',$,(#83362));
#83381=PRESENTATION_STYLE_ASSIGNMENT((#83396));
#83396=SURFACE_STYLE_USAGE(.BOTH.,#83411);
#83411=SURFACE_SIDE_STYLE('',(#83426));
#83426=SURFACE_STYLE_FILL_AREA(#83441);
#83441=FILL_AREA_STYLE('Opaque(190,194,200)',(#83456));
#83456=FILL_AREA_STYLE_COLOUR('Opaque(190,194,200)',#83471);
#83471=COLOUR_RGB('Opaque(190,194,200)', 0.40784314, 0.44705882, 0.49803922);
ENDSEC;
END-ISO-10303-21;
